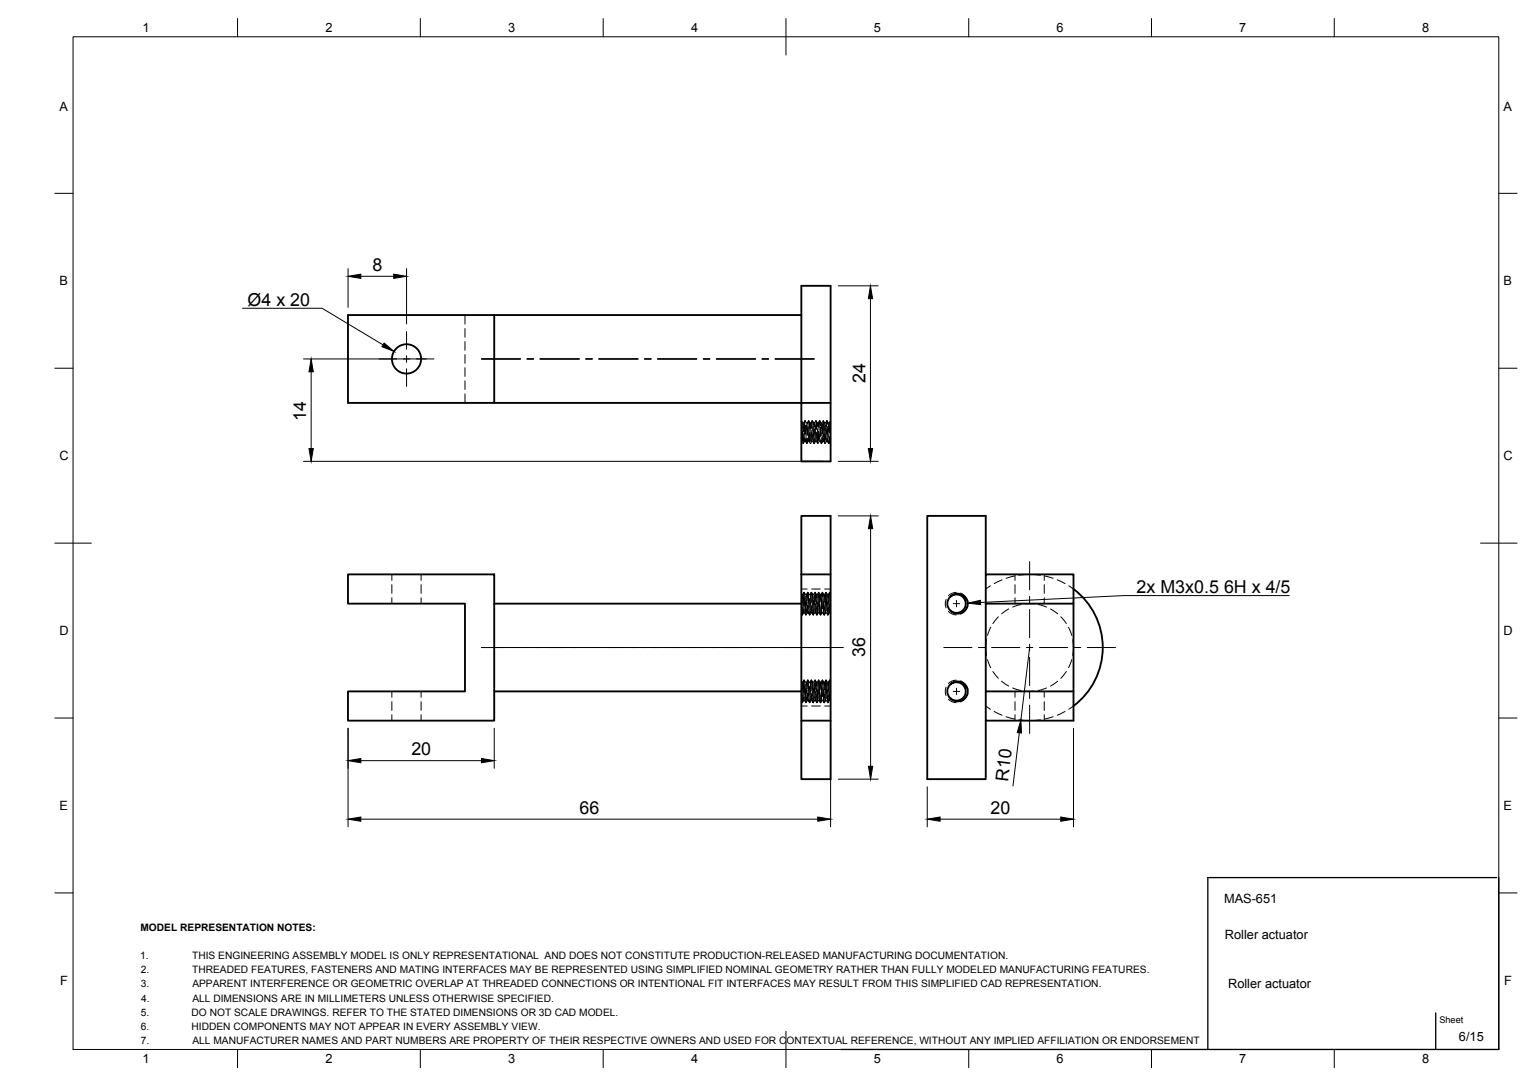
ISO-10303-21;
HEADER;
/* Generated by software containing ST-Developer
 * from STEP Tools, Inc. (www.steptools.com) 
 */

FILE_DESCRIPTION(
/* description */ ('Independent direct-acting normally-closed roller-plunger limit-switch
 CAD. Removable cover, insulated terminal supports, captured bus/conta
ct bridge, native Coil return spring, integral lower travel stop, reus
able instanced hardware and free roller. Manual geometric contact open
ing4mm; no snap-action/contact-force, electrical/current/voltage, envi
ronmental seal, safety-switch, wear, load or life certification. Exter
nal wiring and anchors omitted; fits and application engineering requi
red.'),
/* implementation_level */ '2;1');

FILE_NAME(
/* name */ 'Roller actuator.step',
/* time_stamp */ '2026-11-08T07:32:43-08:00',
/* author */ (''),
/* organization */ (''),
/* preprocessor_version */ 'ST-DEVELOPER v20.2',
/* originating_system */ 'Autodesk Translation Framework v15.17.0.0',
/* authorisation */ '');

FILE_SCHEMA (('AUTOMOTIVE_DESIGN { 1 0 10303 214 3 1 1 }'));
ENDSEC;

DATA;
#10=MECHANICAL_DESIGN_GEOMETRIC_PRESENTATION_REPRESENTATION('',(#179),#36482);
#145=SHAPE_REPRESENTATION_RELATIONSHIP('SRR','None',#36558,#162);
#162=ADVANCED_BREP_SHAPE_REPRESENTATION('',(#196),#36468);
#179=STYLED_ITEM('',(#36652),#196);
#196=MANIFOLD_SOLID_BREP('Body1',#9770);
#218=B_SPLINE_SURFACE_WITH_KNOTS('',3,3,((#21599,#21600,#21601,#21602,#21603,
#21604,#21605,#21606,#21607,#21608,#21609,#21610,#21611,#21612,#21613,#21614,
#21615,#21616,#21617,#21618,#21619,#21620,#21621,#21622,#21623,#21624,#21625,
#21626,#21627,#21628,#21629,#21630,#21631,#21632,#21633,#21634,#21635,#21636,
#21637,#21638,#21639,#21640,#21641,#21642,#21643,#21644,#21645,#21646,#21647,
#21648,#21649,#21650,#21651,#21652,#21653,#21654),(#21655,#21656,#21657,
#21658,#21659,#21660,#21661,#21662,#21663,#21664,#21665,#21666,#21667,#21668,
#21669,#21670,#21671,#21672,#21673,#21674,#21675,#21676,#21677,#21678,#21679,
#21680,#21681,#21682,#21683,#21684,#21685,#21686,#21687,#21688,#21689,#21690,
#21691,#21692,#21693,#21694,#21695,#21696,#21697,#21698,#21699,#21700,#21701,
#21702,#21703,#21704,#21705,#21706,#21707,#21708,#21709,#21710),(#21711,
#21712,#21713,#21714,#21715,#21716,#21717,#21718,#21719,#21720,#21721,#21722,
#21723,#21724,#21725,#21726,#21727,#21728,#21729,#21730,#21731,#21732,#21733,
#21734,#21735,#21736,#21737,#21738,#21739,#21740,#21741,#21742,#21743,#21744,
#21745,#21746,#21747,#21748,#21749,#21750,#21751,#21752,#21753,#21754,#21755,
#21756,#21757,#21758,#21759,#21760,#21761,#21762,#21763,#21764,#21765,#21766),
(#21767,#21768,#21769,#21770,#21771,#21772,#21773,#21774,#21775,#21776,
#21777,#21778,#21779,#21780,#21781,#21782,#21783,#21784,#21785,#21786,#21787,
#21788,#21789,#21790,#21791,#21792,#21793,#21794,#21795,#21796,#21797,#21798,
#21799,#21800,#21801,#21802,#21803,#21804,#21805,#21806,#21807,#21808,#21809,
#21810,#21811,#21812,#21813,#21814,#21815,#21816,#21817,#21818,#21819,#21820,
#21821,#21822)),.UNSPECIFIED.,.F.,.F.,.F.,(4,4),(4,1,1,1,1,1,1,1,1,1,1,
1,1,1,1,1,1,1,1,1,1,1,1,1,1,1,1,1,1,1,1,1,1,1,1,1,1,1,1,1,1,1,1,1,1,1,1,
1,1,1,1,1,1,4),(0.,0.0321584099938621),(11.8553612635793,12.8418906022433,
13.8284199409074,14.8149492795714,15.8014786182354,16.7880079568995,17.7745372955635,
18.7610666342275,19.7475959728915,20.7341253115556,21.7206546502196,22.7071839888836,
23.6937133275477,24.6802426662117,25.6667720048757,26.6533013435398,27.6398306822038,
28.6263600208678,29.6128893595319,30.5994186981959,31.5859480368599,32.5724773755239,
33.559006714188,34.545536052852,35.532065391516,36.5185947301801,37.5051240688441,
38.4916534075081,39.4781827461722,40.4647120848362,41.4512414235002,42.4377707621643,
43.4243001008283,44.4108294394923,45.3973587781563,46.3838881168204,47.3704174554844,
48.3569467941484,49.3434761328125,50.3300054714765,51.3165348101405,52.3030641488046,
53.2895934874686,54.2761228261326,55.2626521647967,56.2491815034607,57.2357108421247,
58.2222401807888,59.2087695194528,60.1952988581168,61.1818281967808,62.1683575354449,
63.1548868741089,64.1414162127729),.UNSPECIFIED.);
#219=B_SPLINE_SURFACE_WITH_KNOTS('',3,3,((#21949,#21950,#21951,#21952,#21953,
#21954,#21955,#21956,#21957,#21958,#21959,#21960,#21961,#21962,#21963,#21964,
#21965,#21966,#21967,#21968,#21969,#21970,#21971,#21972,#21973,#21974,#21975,
#21976,#21977,#21978,#21979,#21980,#21981,#21982,#21983,#21984,#21985,#21986,
#21987,#21988,#21989,#21990,#21991,#21992,#21993,#21994,#21995,#21996,#21997,
#21998,#21999,#22000,#22001,#22002,#22003,#22004),(#22005,#22006,#22007,
#22008,#22009,#22010,#22011,#22012,#22013,#22014,#22015,#22016,#22017,#22018,
#22019,#22020,#22021,#22022,#22023,#22024,#22025,#22026,#22027,#22028,#22029,
#22030,#22031,#22032,#22033,#22034,#22035,#22036,#22037,#22038,#22039,#22040,
#22041,#22042,#22043,#22044,#22045,#22046,#22047,#22048,#22049,#22050,#22051,
#22052,#22053,#22054,#22055,#22056,#22057,#22058,#22059,#22060),(#22061,
#22062,#22063,#22064,#22065,#22066,#22067,#22068,#22069,#22070,#22071,#22072,
#22073,#22074,#22075,#22076,#22077,#22078,#22079,#22080,#22081,#22082,#22083,
#22084,#22085,#22086,#22087,#22088,#22089,#22090,#22091,#22092,#22093,#22094,
#22095,#22096,#22097,#22098,#22099,#22100,#22101,#22102,#22103,#22104,#22105,
#22106,#22107,#22108,#22109,#22110,#22111,#22112,#22113,#22114,#22115,#22116),
(#22117,#22118,#22119,#22120,#22121,#22122,#22123,#22124,#22125,#22126,
#22127,#22128,#22129,#22130,#22131,#22132,#22133,#22134,#22135,#22136,#22137,
#22138,#22139,#22140,#22141,#22142,#22143,#22144,#22145,#22146,#22147,#22148,
#22149,#22150,#22151,#22152,#22153,#22154,#22155,#22156,#22157,#22158,#22159,
#22160,#22161,#22162,#22163,#22164,#22165,#22166,#22167,#22168,#22169,#22170,
#22171,#22172)),.UNSPECIFIED.,.F.,.F.,.F.,(4,4),(4,1,1,1,1,1,1,1,1,1,1,
1,1,1,1,1,1,1,1,1,1,1,1,1,1,1,1,1,1,1,1,1,1,1,1,1,1,1,1,1,1,1,1,1,1,1,1,
1,1,1,1,1,1,4),(0.,0.0321584099938621),(14.3984001269718,15.3849294656359,
16.3714588042999,17.3579881429639,18.344517481628,19.331046820292,20.317576158956,
21.30410549762,22.2906348362841,23.2771641749481,24.2636935136121,25.2502228522762,
26.2367521909402,27.2232815296042,28.2098108682683,29.1963402069323,30.1828695455963,
31.1693988842604,32.1559282229244,33.1424575615884,34.1289869002524,35.1155162389165,
36.1020455775805,37.0885749162445,38.0751042549086,39.0616335935726,40.0481629322366,
41.0346922709007,42.0212216095647,43.0077509482287,43.9942802868928,44.9808096255568,
45.9673389642208,46.9538683028848,47.9403976415489,48.9269269802129,49.9134563188769,
50.899985657541,51.886514996205,52.873044334869,53.8595736735331,54.8461030121971,
55.8326323508611,56.8191616895251,57.8056910281892,58.7922203668532,59.7787497055172,
60.7652790441813,61.7518083828453,62.7383377215093,63.7248670601734,64.7113963988374,
65.6979257375014,66.6844550761655),.UNSPECIFIED.);
#220=B_SPLINE_SURFACE_WITH_KNOTS('',3,3,((#22435,#22436,#22437,#22438,#22439,
#22440,#22441,#22442,#22443,#22444,#22445,#22446,#22447,#22448,#22449,#22450,
#22451,#22452,#22453,#22454,#22455,#22456,#22457,#22458,#22459,#22460,#22461,
#22462,#22463,#22464,#22465,#22466,#22467,#22468,#22469,#22470,#22471,#22472,
#22473,#22474,#22475,#22476,#22477,#22478,#22479,#22480,#22481,#22482,#22483,
#22484,#22485,#22486,#22487,#22488,#22489,#22490),(#22491,#22492,#22493,
#22494,#22495,#22496,#22497,#22498,#22499,#22500,#22501,#22502,#22503,#22504,
#22505,#22506,#22507,#22508,#22509,#22510,#22511,#22512,#22513,#22514,#22515,
#22516,#22517,#22518,#22519,#22520,#22521,#22522,#22523,#22524,#22525,#22526,
#22527,#22528,#22529,#22530,#22531,#22532,#22533,#22534,#22535,#22536,#22537,
#22538,#22539,#22540,#22541,#22542,#22543,#22544,#22545,#22546),(#22547,
#22548,#22549,#22550,#22551,#22552,#22553,#22554,#22555,#22556,#22557,#22558,
#22559,#22560,#22561,#22562,#22563,#22564,#22565,#22566,#22567,#22568,#22569,
#22570,#22571,#22572,#22573,#22574,#22575,#22576,#22577,#22578,#22579,#22580,
#22581,#22582,#22583,#22584,#22585,#22586,#22587,#22588,#22589,#22590,#22591,
#22592,#22593,#22594,#22595,#22596,#22597,#22598,#22599,#22600,#22601,#22602),
(#22603,#22604,#22605,#22606,#22607,#22608,#22609,#22610,#22611,#22612,
#22613,#22614,#22615,#22616,#22617,#22618,#22619,#22620,#22621,#22622,#22623,
#22624,#22625,#22626,#22627,#22628,#22629,#22630,#22631,#22632,#22633,#22634,
#22635,#22636,#22637,#22638,#22639,#22640,#22641,#22642,#22643,#22644,#22645,
#22646,#22647,#22648,#22649,#22650,#22651,#22652,#22653,#22654,#22655,#22656,
#22657,#22658)),.UNSPECIFIED.,.F.,.F.,.F.,(4,4),(4,1,1,1,1,1,1,1,1,1,1,
1,1,1,1,1,1,1,1,1,1,1,1,1,1,1,1,1,1,1,1,1,1,1,1,1,1,1,1,1,1,1,1,1,1,1,1,
1,1,1,1,1,1,4),(0.,0.0321584099938621),(11.8553612635793,12.8418906022433,
13.8284199409074,14.8149492795714,15.8014786182354,16.7880079568995,17.7745372955635,
18.7610666342275,19.7475959728915,20.7341253115556,21.7206546502196,22.7071839888836,
23.6937133275477,24.6802426662117,25.6667720048757,26.6533013435398,27.6398306822038,
28.6263600208678,29.6128893595319,30.5994186981959,31.5859480368599,32.5724773755239,
33.559006714188,34.545536052852,35.532065391516,36.5185947301801,37.5051240688441,
38.4916534075081,39.4781827461722,40.4647120848362,41.4512414235002,42.4377707621643,
43.4243001008283,44.4108294394923,45.3973587781563,46.3838881168204,47.3704174554844,
48.3569467941484,49.3434761328125,50.3300054714765,51.3165348101405,52.3030641488046,
53.2895934874686,54.2761228261326,55.2626521647967,56.2491815034607,57.2357108421247,
58.2222401807888,59.2087695194528,60.1952988581168,61.1818281967808,62.1683575354449,
63.1548868741089,64.1414162127729),.UNSPECIFIED.);
#221=B_SPLINE_SURFACE_WITH_KNOTS('',3,3,((#22733,#22734,#22735,#22736,#22737,
#22738,#22739,#22740,#22741,#22742,#22743,#22744,#22745,#22746,#22747,#22748,
#22749,#22750,#22751,#22752,#22753,#22754,#22755,#22756,#22757,#22758,#22759,
#22760,#22761,#22762,#22763,#22764,#22765,#22766,#22767,#22768,#22769,#22770,
#22771,#22772,#22773,#22774,#22775,#22776,#22777,#22778,#22779,#22780,#22781,
#22782,#22783,#22784,#22785,#22786,#22787,#22788),(#22789,#22790,#22791,
#22792,#22793,#22794,#22795,#22796,#22797,#22798,#22799,#22800,#22801,#22802,
#22803,#22804,#22805,#22806,#22807,#22808,#22809,#22810,#22811,#22812,#22813,
#22814,#22815,#22816,#22817,#22818,#22819,#22820,#22821,#22822,#22823,#22824,
#22825,#22826,#22827,#22828,#22829,#22830,#22831,#22832,#22833,#22834,#22835,
#22836,#22837,#22838,#22839,#22840,#22841,#22842,#22843,#22844),(#22845,
#22846,#22847,#22848,#22849,#22850,#22851,#22852,#22853,#22854,#22855,#22856,
#22857,#22858,#22859,#22860,#22861,#22862,#22863,#22864,#22865,#22866,#22867,
#22868,#22869,#22870,#22871,#22872,#22873,#22874,#22875,#22876,#22877,#22878,
#22879,#22880,#22881,#22882,#22883,#22884,#22885,#22886,#22887,#22888,#22889,
#22890,#22891,#22892,#22893,#22894,#22895,#22896,#22897,#22898,#22899,#22900),
(#22901,#22902,#22903,#22904,#22905,#22906,#22907,#22908,#22909,#22910,
#22911,#22912,#22913,#22914,#22915,#22916,#22917,#22918,#22919,#22920,#22921,
#22922,#22923,#22924,#22925,#22926,#22927,#22928,#22929,#22930,#22931,#22932,
#22933,#22934,#22935,#22936,#22937,#22938,#22939,#22940,#22941,#22942,#22943,
#22944,#22945,#22946,#22947,#22948,#22949,#22950,#22951,#22952,#22953,#22954,
#22955,#22956)),.UNSPECIFIED.,.F.,.F.,.F.,(4,4),(4,1,1,1,1,1,1,1,1,1,1,
1,1,1,1,1,1,1,1,1,1,1,1,1,1,1,1,1,1,1,1,1,1,1,1,1,1,1,1,1,1,1,1,1,1,1,1,
1,1,1,1,1,1,4),(0.,0.0321584099938621),(14.3984001269718,15.3849294656359,
16.3714588042999,17.3579881429639,18.344517481628,19.331046820292,20.317576158956,
21.30410549762,22.2906348362841,23.2771641749481,24.2636935136121,25.2502228522762,
26.2367521909402,27.2232815296042,28.2098108682683,29.1963402069323,30.1828695455963,
31.1693988842604,32.1559282229244,33.1424575615884,34.1289869002524,35.1155162389165,
36.1020455775805,37.0885749162445,38.0751042549086,39.0616335935726,40.0481629322366,
41.0346922709007,42.0212216095647,43.0077509482287,43.9942802868928,44.9808096255568,
45.9673389642208,46.9538683028848,47.9403976415489,48.9269269802129,49.9134563188769,
50.899985657541,51.886514996205,52.873044334869,53.8595736735331,54.8461030121971,
55.8326323508611,56.8191616895251,57.8056910281892,58.7922203668532,59.7787497055172,
60.7652790441813,61.7518083828453,62.7383377215093,63.7248670601734,64.7113963988374,
65.6979257375014,66.6844550761655),.UNSPECIFIED.);
#267=FACE_BOUND('',#1222,.T.);
#268=FACE_BOUND('',#1223,.T.);
#269=FACE_BOUND('',#1232,.T.);
#270=FACE_BOUND('',#1237,.T.);
#271=FACE_BOUND('',#1243,.T.);
#272=FACE_BOUND('',#1245,.T.);
#273=FACE_BOUND('',#1254,.T.);
#274=FACE_BOUND('',#1255,.T.);
#275=FACE_BOUND('',#1256,.T.);
#342=PLANE('',#10249);
#343=PLANE('',#10260);
#344=PLANE('',#10261);
#345=PLANE('',#10262);
#346=PLANE('',#10263);
#347=PLANE('',#10264);
#348=PLANE('',#10265);
#349=PLANE('',#10266);
#350=PLANE('',#10268);
#351=PLANE('',#10271);
#352=PLANE('',#10272);
#353=PLANE('',#10273);
#354=PLANE('',#10274);
#355=PLANE('',#10275);
#356=PLANE('',#10276);
#357=PLANE('',#10277);
#358=PLANE('',#10278);
#359=PLANE('',#10283);
#616=FACE_OUTER_BOUND('',#1186,.T.);
#617=FACE_OUTER_BOUND('',#1187,.T.);
#618=FACE_OUTER_BOUND('',#1188,.T.);
#619=FACE_OUTER_BOUND('',#1189,.T.);
#620=FACE_OUTER_BOUND('',#1190,.T.);
#621=FACE_OUTER_BOUND('',#1191,.T.);
#622=FACE_OUTER_BOUND('',#1192,.T.);
#623=FACE_OUTER_BOUND('',#1193,.T.);
#624=FACE_OUTER_BOUND('',#1194,.T.);
#625=FACE_OUTER_BOUND('',#1195,.T.);
#626=FACE_OUTER_BOUND('',#1196,.T.);
#627=FACE_OUTER_BOUND('',#1197,.T.);
#628=FACE_OUTER_BOUND('',#1198,.T.);
#629=FACE_OUTER_BOUND('',#1199,.T.);
#630=FACE_OUTER_BOUND('',#1200,.T.);
#631=FACE_OUTER_BOUND('',#1201,.T.);
#632=FACE_OUTER_BOUND('',#1202,.T.);
#633=FACE_OUTER_BOUND('',#1203,.T.);
#634=FACE_OUTER_BOUND('',#1204,.T.);
#635=FACE_OUTER_BOUND('',#1205,.T.);
#636=FACE_OUTER_BOUND('',#1206,.T.);
#637=FACE_OUTER_BOUND('',#1207,.T.);
#638=FACE_OUTER_BOUND('',#1208,.T.);
#639=FACE_OUTER_BOUND('',#1209,.T.);
#640=FACE_OUTER_BOUND('',#1210,.T.);
#641=FACE_OUTER_BOUND('',#1211,.T.);
#642=FACE_OUTER_BOUND('',#1212,.T.);
#643=FACE_OUTER_BOUND('',#1213,.T.);
#644=FACE_OUTER_BOUND('',#1214,.T.);
#645=FACE_OUTER_BOUND('',#1215,.T.);
#646=FACE_OUTER_BOUND('',#1216,.T.);
#647=FACE_OUTER_BOUND('',#1217,.T.);
#648=FACE_OUTER_BOUND('',#1218,.T.);
#649=FACE_OUTER_BOUND('',#1219,.T.);
#650=FACE_OUTER_BOUND('',#1220,.T.);
#651=FACE_OUTER_BOUND('',#1221,.T.);
#652=FACE_OUTER_BOUND('',#1224,.T.);
#653=FACE_OUTER_BOUND('',#1225,.T.);
#654=FACE_OUTER_BOUND('',#1226,.T.);
#655=FACE_OUTER_BOUND('',#1227,.T.);
#656=FACE_OUTER_BOUND('',#1228,.T.);
#657=FACE_OUTER_BOUND('',#1229,.T.);
#658=FACE_OUTER_BOUND('',#1230,.T.);
#659=FACE_OUTER_BOUND('',#1231,.T.);
#660=FACE_OUTER_BOUND('',#1233,.T.);
#661=FACE_OUTER_BOUND('',#1234,.T.);
#662=FACE_OUTER_BOUND('',#1235,.T.);
#663=FACE_OUTER_BOUND('',#1236,.T.);
#664=FACE_OUTER_BOUND('',#1238,.T.);
#665=FACE_OUTER_BOUND('',#1239,.T.);
#666=FACE_OUTER_BOUND('',#1240,.T.);
#667=FACE_OUTER_BOUND('',#1241,.T.);
#668=FACE_OUTER_BOUND('',#1242,.T.);
#669=FACE_OUTER_BOUND('',#1244,.T.);
#670=FACE_OUTER_BOUND('',#1246,.T.);
#671=FACE_OUTER_BOUND('',#1247,.T.);
#672=FACE_OUTER_BOUND('',#1248,.T.);
#673=FACE_OUTER_BOUND('',#1249,.T.);
#674=FACE_OUTER_BOUND('',#1250,.T.);
#675=FACE_OUTER_BOUND('',#1251,.T.);
#676=FACE_OUTER_BOUND('',#1252,.T.);
#677=FACE_OUTER_BOUND('',#1253,.T.);
#1186=EDGE_LOOP('',(#6952,#6953,#6954,#6955));
#1187=EDGE_LOOP('',(#6956,#6957,#6958,#6959));
#1188=EDGE_LOOP('',(#6960,#6961,#6962,#6963));
#1189=EDGE_LOOP('',(#6964,#6965,#6966,#6967));
#1190=EDGE_LOOP('',(#6968,#6969,#6970,#6971));
#1191=EDGE_LOOP('',(#6972,#6973,#6974,#6975));
#1192=EDGE_LOOP('',(#6976,#6977,#6978,#6979));
#1193=EDGE_LOOP('',(#6980,#6981,#6982,#6983));
#1194=EDGE_LOOP('',(#6984,#6985,#6986,#6987));
#1195=EDGE_LOOP('',(#6988,#6989,#6990,#6991));
#1196=EDGE_LOOP('',(#6992,#6993,#6994,#6995));
#1197=EDGE_LOOP('',(#6996,#6997,#6998,#6999));
#1198=EDGE_LOOP('',(#7000,#7001,#7002,#7003));
#1199=EDGE_LOOP('',(#7004,#7005,#7006,#7007));
#1200=EDGE_LOOP('',(#7008,#7009,#7010,#7011));
#1201=EDGE_LOOP('',(#7012,#7013,#7014,#7015));
#1202=EDGE_LOOP('',(#7016,#7017,#7018,#7019));
#1203=EDGE_LOOP('',(#7020,#7021,#7022,#7023));
#1204=EDGE_LOOP('',(#7024,#7025,#7026,#7027));
#1205=EDGE_LOOP('',(#7028,#7029,#7030,#7031));
#1206=EDGE_LOOP('',(#7032,#7033,#7034,#7035));
#1207=EDGE_LOOP('',(#7036,#7037,#7038,#7039));
#1208=EDGE_LOOP('',(#7040,#7041,#7042,#7043));
#1209=EDGE_LOOP('',(#7044,#7045,#7046,#7047));
#1210=EDGE_LOOP('',(#7048,#7049,#7050,#7051));
#1211=EDGE_LOOP('',(#7052,#7053,#7054,#7055));
#1212=EDGE_LOOP('',(#7056,#7057,#7058,#7059));
#1213=EDGE_LOOP('',(#7060,#7061,#7062,#7063));
#1214=EDGE_LOOP('',(#7064,#7065,#7066,#7067));
#1215=EDGE_LOOP('',(#7068,#7069,#7070,#7071));
#1216=EDGE_LOOP('',(#7072,#7073,#7074,#7075));
#1217=EDGE_LOOP('',(#7076,#7077,#7078,#7079));
#1218=EDGE_LOOP('',(#7080,#7081,#7082,#7083));
#1219=EDGE_LOOP('',(#7084,#7085,#7086,#7087,#7088,#7089,#7090,#7091,#7092,
#7093,#7094,#7095,#7096,#7097,#7098,#7099,#7100,#7101,#7102,#7103));
#1220=EDGE_LOOP('',(#7104,#7105,#7106,#7107,#7108,#7109,#7110,#7111,#7112,
#7113,#7114,#7115,#7116,#7117,#7118,#7119,#7120,#7121,#7122,#7123));
#1221=EDGE_LOOP('',(#7124,#7125,#7126,#7127,#7128,#7129));
#1222=EDGE_LOOP('',(#7130,#7131,#7132,#7133));
#1223=EDGE_LOOP('',(#7134,#7135,#7136,#7137));
#1224=EDGE_LOOP('',(#7138,#7139,#7140,#7141));
#1225=EDGE_LOOP('',(#7142,#7143,#7144,#7145,#7146,#7147,#7148,#7149,#7150,
#7151,#7152,#7153,#7154,#7155,#7156,#7157,#7158,#7159,#7160,#7161));
#1226=EDGE_LOOP('',(#7162,#7163,#7164,#7165,#7166,#7167,#7168,#7169,#7170,
#7171,#7172,#7173,#7174,#7175,#7176,#7177,#7178,#7179,#7180,#7181));
#1227=EDGE_LOOP('',(#7182,#7183,#7184,#7185));
#1228=EDGE_LOOP('',(#7186,#7187,#7188,#7189));
#1229=EDGE_LOOP('',(#7190,#7191,#7192,#7193));
#1230=EDGE_LOOP('',(#7194,#7195,#7196,#7197));
#1231=EDGE_LOOP('',(#7198,#7199,#7200,#7201));
#1232=EDGE_LOOP('',(#7202));
#1233=EDGE_LOOP('',(#7203,#7204,#7205,#7206));
#1234=EDGE_LOOP('',(#7207,#7208,#7209,#7210,#7211,#7212,#7213,#7214,#7215));
#1235=EDGE_LOOP('',(#7216,#7217,#7218,#7219));
#1236=EDGE_LOOP('',(#7220,#7221,#7222,#7223));
#1237=EDGE_LOOP('',(#7224));
#1238=EDGE_LOOP('',(#7225,#7226,#7227,#7228));
#1239=EDGE_LOOP('',(#7229,#7230,#7231,#7232));
#1240=EDGE_LOOP('',(#7233,#7234,#7235,#7236,#7237));
#1241=EDGE_LOOP('',(#7238,#7239,#7240,#7241,#7242,#7243,#7244,#7245,#7246));
#1242=EDGE_LOOP('',(#7247,#7248,#7249,#7250));
#1243=EDGE_LOOP('',(#7251));
#1244=EDGE_LOOP('',(#7252,#7253,#7254,#7255));
#1245=EDGE_LOOP('',(#7256));
#1246=EDGE_LOOP('',(#7257,#7258,#7259,#7260));
#1247=EDGE_LOOP('',(#7261,#7262,#7263,#7264));
#1248=EDGE_LOOP('',(#7265,#7266,#7267,#7268));
#1249=EDGE_LOOP('',(#7269,#7270,#7271,#7272));
#1250=EDGE_LOOP('',(#7273,#7274,#7275,#7276));
#1251=EDGE_LOOP('',(#7277,#7278,#7279,#7280));
#1252=EDGE_LOOP('',(#7281,#7282,#7283,#7284,#7285,#7286));
#1253=EDGE_LOOP('',(#7287,#7288,#7289,#7290,#7291,#7292));
#1254=EDGE_LOOP('',(#7293,#7294,#7295,#7296));
#1255=EDGE_LOOP('',(#7297,#7298,#7299,#7300));
#1256=EDGE_LOOP('',(#7301));
#1644=CIRCLE('',#10209,0.12645);
#1645=CIRCLE('',#10217,0.12645);
#1646=CIRCLE('',#10219,0.12645);
#1647=CIRCLE('',#10227,0.12645);
#1648=CIRCLE('',#10229,0.1543);
#1649=CIRCLE('',#10237,0.1543);
#1650=CIRCLE('',#10239,0.1543);
#1651=CIRCLE('',#10247,0.1543);
#1652=CIRCLE('',#10250,1.);
#1653=CIRCLE('',#10255,0.2);
#1654=CIRCLE('',#10256,0.2);
#1655=CIRCLE('',#10258,0.2);
#1656=CIRCLE('',#10259,0.2);
#1657=CIRCLE('',#10267,0.6);
#1658=CIRCLE('',#10269,0.6);
#1659=CIRCLE('',#10270,0.6);
#1660=CIRCLE('',#10280,1.);
#1661=CIRCLE('',#10282,0.6);
#1974=B_SPLINE_CURVE_WITH_KNOTS('',3,(#20484,#20485,#20486,#20487),
 .UNSPECIFIED.,.F.,.F.,(4,4),(51.5750455984138,52.2860549491936),
 .UNSPECIFIED.);
#1975=B_SPLINE_CURVE_WITH_KNOTS('',3,(#20490,#20491,#20492,#20493,#20494,
#20495,#20496,#20497,#20498,#20499),.UNSPECIFIED.,.F.,.F.,(4,3,3,4),(-50.2654824574367,
-49.3264669332015,-48.3399375945375,-47.8348991546268),.UNSPECIFIED.);
#1976=B_SPLINE_CURVE_WITH_KNOTS('',3,(#20504,#20505,#20506,#20507,#20508,
#20509,#20510,#20511,#20512,#20513,#20514,#20515,#20516,#20517,#20518,#20519,
#20520,#20521,#20522,#20523,#20524,#20525,#20526,#20527,#20528),
 .UNSPECIFIED.,.F.,.F.,(4,3,3,3,3,3,3,3,4),(45.2918602912342,45.3803495785454,
46.3668789172094,47.3534082558735,48.3399375945375,49.3264669332015,50.3129962718656,
51.2995256105296,51.5750455984138),.UNSPECIFIED.);
#1977=B_SPLINE_CURVE_WITH_KNOTS('',3,(#20529,#20530,#20531,#20532,#20533,
#20534,#20535,#20536,#20537,#20538,#20539,#20540,#20541,#20542,#20543,#20544,
#20545,#20546,#20547,#20548,#20549,#20550),.UNSPECIFIED.,.F.,.F.,(4,3,3,
3,3,3,3,4),(-47.8348991546268,-47.3534082558735,-46.3668789172095,-45.3803495785454,
-44.3938202398814,-43.4072909012174,-42.4207615625533,-41.5517138474472),
 .UNSPECIFIED.);
#1978=B_SPLINE_CURVE_WITH_KNOTS('',3,(#20555,#20556,#20557,#20558,#20559,
#20560,#20561,#20562,#20563,#20564,#20565,#20566,#20567,#20568,#20569,#20570,
#20571,#20572,#20573,#20574,#20575,#20576),.UNSPECIFIED.,.F.,.F.,(4,3,3,
3,3,3,3,4),(39.0086749840546,39.4611735465612,40.4477028852253,41.4342322238893,
42.4207615625533,43.4072909012174,44.3938202398814,45.2918602912342),
 .UNSPECIFIED.);
#1979=B_SPLINE_CURVE_WITH_KNOTS('',3,(#20577,#20578,#20579,#20580,#20581,
#20582,#20583,#20584,#20585,#20586,#20587,#20588,#20589,#20590,#20591,#20592,
#20593,#20594,#20595,#20596,#20597,#20598,#20599,#20600,#20601),
 .UNSPECIFIED.,.F.,.F.,(4,3,3,3,3,3,3,3,4),(-41.5517138474472,-41.4342322238893,
-40.4477028852253,-39.4611735465612,-38.4746442078972,-37.4881148692332,
-36.5015855305691,-35.5150561919051,-35.2685285402676),.UNSPECIFIED.);
#1980=B_SPLINE_CURVE_WITH_KNOTS('',3,(#20606,#20607,#20608,#20609,#20610,
#20611,#20612,#20613,#20614,#20615,#20616,#20617,#20618,#20619,#20620,#20621,
#20622,#20623,#20624,#20625,#20626,#20627),.UNSPECIFIED.,.F.,.F.,(4,3,3,
3,3,3,3,4),(32.725489676875,33.541997514577,34.5285268532411,35.5150561919051,
36.5015855305691,37.4881148692332,38.4746442078972,39.0086749840546),
 .UNSPECIFIED.);
#1981=B_SPLINE_CURVE_WITH_KNOTS('',3,(#20628,#20629,#20630,#20631,#20632,
#20633,#20634,#20635,#20636,#20637,#20638,#20639,#20640,#20641,#20642,#20643,
#20644,#20645,#20646,#20647,#20648,#20649),.UNSPECIFIED.,.F.,.F.,(4,3,3,
3,3,3,3,4),(-35.2685285402676,-34.5285268532411,-33.541997514577,-32.555468175913,
-31.568938837249,-30.582409498585,-29.5958801599209,-28.985343233088),
 .UNSPECIFIED.);
#1982=B_SPLINE_CURVE_WITH_KNOTS('',3,(#20654,#20655,#20656,#20657,#20658,
#20659,#20660,#20661,#20662,#20663,#20664,#20665,#20666,#20667,#20668,#20669,
#20670,#20671,#20672,#20673,#20674,#20675,#20676,#20677,#20678),
 .UNSPECIFIED.,.F.,.F.,(4,3,3,3,3,3,3,3,4),(26.4423043696954,26.6362921439288,
27.6228214825929,28.6093508212569,29.5958801599209,30.582409498585,31.568938837249,
32.555468175913,32.725489676875),.UNSPECIFIED.);
#1983=B_SPLINE_CURVE_WITH_KNOTS('',3,(#20679,#20680,#20681,#20682,#20683,
#20684,#20685,#20686,#20687,#20688,#20689,#20690,#20691,#20692,#20693,#20694,
#20695,#20696,#20697,#20698,#20699,#20700),.UNSPECIFIED.,.F.,.F.,(4,3,3,
3,3,3,3,4),(-28.985343233088,-28.6093508212569,-27.6228214825929,-26.6362921439288,
-25.6497628052648,-24.6632334666008,-23.6767041279367,-22.7021579259084),
 .UNSPECIFIED.);
#1984=B_SPLINE_CURVE_WITH_KNOTS('',3,(#20705,#20706,#20707,#20708,#20709,
#20710,#20711,#20712,#20713,#20714,#20715,#20716,#20717,#20718,#20719,#20720,
#20721,#20722,#20723,#20724,#20725,#20726),.UNSPECIFIED.,.F.,.F.,(4,3,3,
3,3,3,3,4),(20.1591190625159,20.7171161119446,21.7036454506087,22.6901747892727,
23.6767041279367,24.6632334666008,25.6497628052648,26.4423043696954),
 .UNSPECIFIED.);
#1985=B_SPLINE_CURVE_WITH_KNOTS('',3,(#20727,#20728,#20729,#20730,#20731,
#20732,#20733,#20734,#20735,#20736,#20737,#20738,#20739,#20740,#20741,#20742,
#20743,#20744,#20745,#20746,#20747,#20748,#20749,#20750,#20751),
 .UNSPECIFIED.,.F.,.F.,(4,3,3,3,3,3,3,3,4),(-22.7021579259084,-22.6901747892727,
-21.7036454506087,-20.7171161119446,-19.7305867732806,-18.7440574346166,
-17.7575280959526,-16.7709987572885,-16.4189726187288),.UNSPECIFIED.);
#1986=B_SPLINE_CURVE_WITH_KNOTS('',3,(#20756,#20757,#20758,#20759,#20760,
#20761,#20762,#20763,#20764,#20765,#20766,#20767,#20768,#20769,#20770,#20771,
#20772,#20773,#20774,#20775,#20776,#20777),.UNSPECIFIED.,.F.,.F.,(4,3,3,
3,3,3,3,4),(13.8759337553363,14.7979400799605,15.7844694186245,16.7709987572885,
17.7575280959526,18.7440574346166,19.7305867732806,20.1591190625159),
 .UNSPECIFIED.);
#1987=B_SPLINE_CURVE_WITH_KNOTS('',3,(#20778,#20779,#20780,#20781,#20782,
#20783,#20784,#20785,#20786,#20787,#20788,#20789,#20790,#20791,#20792,#20793,
#20794,#20795,#20796,#20797,#20798,#20799),.UNSPECIFIED.,.F.,.F.,(4,3,3,
3,3,3,3,4),(-16.4189726187288,-15.7844694186245,-14.7979400799605,-13.8114107412964,
-12.8248814026324,-11.8383520639684,-10.8518227253043,-10.1357873115492),
 .UNSPECIFIED.);
#1988=B_SPLINE_CURVE_WITH_KNOTS('',3,(#20805,#20806,#20807,#20808,#20809,
#20810,#20811,#20812,#20813,#20814,#20815,#20816,#20817),.UNSPECIFIED.,
 .F.,.F.,(4,3,3,3,4),(-3.85260200436966,-2.95958801599209,-1.97305867732806,
-0.986529338664031,0.),.UNSPECIFIED.);
#1989=B_SPLINE_CURVE_WITH_KNOTS('',3,(#20820,#20821,#20822,#20823,#20824,
#20825,#20826,#20827,#20828,#20829,#20830,#20831,#20832,#20833,#20834,#20835,
#20836,#20837,#20838),.UNSPECIFIED.,.F.,.F.,(4,3,3,3,3,3,4),(2.0205724917569,
2.95958801599209,3.94611735465613,4.93264669332016,5.91917603198418,6.90570537064821,
7.5927484481567),.UNSPECIFIED.);
#1990=B_SPLINE_CURVE_WITH_KNOTS('',3,(#20844,#20845,#20846,#20847),
 .UNSPECIFIED.,.F.,.F.,(4,4),(51.5750455984138,52.2860549491936),
 .UNSPECIFIED.);
#1991=B_SPLINE_CURVE_WITH_KNOTS('',3,(#20850,#20851,#20852,#20853,#20854,
#20855,#20856,#20857,#20858,#20859),.UNSPECIFIED.,.F.,.F.,(4,3,3,4),(-50.2654824574367,
-49.3264669332015,-48.3399375945375,-47.8348991546268),.UNSPECIFIED.);
#1992=B_SPLINE_CURVE_WITH_KNOTS('',3,(#20864,#20865,#20866,#20867,#20868,
#20869,#20870,#20871,#20872,#20873,#20874,#20875,#20876,#20877,#20878,#20879,
#20880,#20881,#20882,#20883,#20884,#20885,#20886,#20887,#20888),
 .UNSPECIFIED.,.F.,.F.,(4,3,3,3,3,3,3,3,4),(45.2918602912342,45.3803495785454,
46.3668789172094,47.3534082558735,48.3399375945375,49.3264669332015,50.3129962718656,
51.2995256105296,51.5750455984138),.UNSPECIFIED.);
#1993=B_SPLINE_CURVE_WITH_KNOTS('',3,(#20889,#20890,#20891,#20892,#20893,
#20894,#20895,#20896,#20897,#20898,#20899,#20900,#20901,#20902,#20903,#20904,
#20905,#20906,#20907,#20908,#20909,#20910),.UNSPECIFIED.,.F.,.F.,(4,3,3,
3,3,3,3,4),(-47.8348991546268,-47.3534082558735,-46.3668789172095,-45.3803495785454,
-44.3938202398814,-43.4072909012174,-42.4207615625533,-41.5517138474472),
 .UNSPECIFIED.);
#1994=B_SPLINE_CURVE_WITH_KNOTS('',3,(#20915,#20916,#20917,#20918,#20919,
#20920,#20921,#20922,#20923,#20924,#20925,#20926,#20927,#20928,#20929,#20930,
#20931,#20932,#20933,#20934,#20935,#20936),.UNSPECIFIED.,.F.,.F.,(4,3,3,
3,3,3,3,4),(39.0086749840546,39.4611735465612,40.4477028852253,41.4342322238893,
42.4207615625533,43.4072909012174,44.3938202398814,45.2918602912342),
 .UNSPECIFIED.);
#1995=B_SPLINE_CURVE_WITH_KNOTS('',3,(#20937,#20938,#20939,#20940,#20941,
#20942,#20943,#20944,#20945,#20946,#20947,#20948,#20949,#20950,#20951,#20952,
#20953,#20954,#20955,#20956,#20957,#20958,#20959,#20960,#20961),
 .UNSPECIFIED.,.F.,.F.,(4,3,3,3,3,3,3,3,4),(-41.5517138474472,-41.4342322238893,
-40.4477028852253,-39.4611735465612,-38.4746442078972,-37.4881148692332,
-36.5015855305691,-35.5150561919051,-35.2685285402676),.UNSPECIFIED.);
#1996=B_SPLINE_CURVE_WITH_KNOTS('',3,(#20966,#20967,#20968,#20969,#20970,
#20971,#20972,#20973,#20974,#20975,#20976,#20977,#20978,#20979,#20980,#20981,
#20982,#20983,#20984,#20985,#20986,#20987),.UNSPECIFIED.,.F.,.F.,(4,3,3,
3,3,3,3,4),(32.725489676875,33.541997514577,34.5285268532411,35.5150561919051,
36.5015855305691,37.4881148692332,38.4746442078972,39.0086749840546),
 .UNSPECIFIED.);
#1997=B_SPLINE_CURVE_WITH_KNOTS('',3,(#20988,#20989,#20990,#20991,#20992,
#20993,#20994,#20995,#20996,#20997,#20998,#20999,#21000,#21001,#21002,#21003,
#21004,#21005,#21006,#21007,#21008,#21009),.UNSPECIFIED.,.F.,.F.,(4,3,3,
3,3,3,3,4),(-35.2685285402676,-34.5285268532411,-33.541997514577,-32.555468175913,
-31.568938837249,-30.582409498585,-29.5958801599209,-28.985343233088),
 .UNSPECIFIED.);
#1998=B_SPLINE_CURVE_WITH_KNOTS('',3,(#21014,#21015,#21016,#21017,#21018,
#21019,#21020,#21021,#21022,#21023,#21024,#21025,#21026,#21027,#21028,#21029,
#21030,#21031,#21032,#21033,#21034,#21035,#21036,#21037,#21038),
 .UNSPECIFIED.,.F.,.F.,(4,3,3,3,3,3,3,3,4),(26.4423043696954,26.6362921439288,
27.6228214825929,28.6093508212569,29.5958801599209,30.582409498585,31.568938837249,
32.555468175913,32.725489676875),.UNSPECIFIED.);
#1999=B_SPLINE_CURVE_WITH_KNOTS('',3,(#21039,#21040,#21041,#21042,#21043,
#21044,#21045,#21046,#21047,#21048,#21049,#21050,#21051,#21052,#21053,#21054,
#21055,#21056,#21057,#21058,#21059,#21060),.UNSPECIFIED.,.F.,.F.,(4,3,3,
3,3,3,3,4),(-28.985343233088,-28.6093508212569,-27.6228214825929,-26.6362921439288,
-25.6497628052648,-24.6632334666008,-23.6767041279367,-22.7021579259084),
 .UNSPECIFIED.);
#2000=B_SPLINE_CURVE_WITH_KNOTS('',3,(#21065,#21066,#21067,#21068,#21069,
#21070,#21071,#21072,#21073,#21074,#21075,#21076,#21077,#21078,#21079,#21080,
#21081,#21082,#21083,#21084,#21085,#21086),.UNSPECIFIED.,.F.,.F.,(4,3,3,
3,3,3,3,4),(20.1591190625159,20.7171161119446,21.7036454506087,22.6901747892727,
23.6767041279367,24.6632334666008,25.6497628052648,26.4423043696954),
 .UNSPECIFIED.);
#2001=B_SPLINE_CURVE_WITH_KNOTS('',3,(#21087,#21088,#21089,#21090,#21091,
#21092,#21093,#21094,#21095,#21096,#21097,#21098,#21099,#21100,#21101,#21102,
#21103,#21104,#21105,#21106,#21107,#21108,#21109,#21110,#21111),
 .UNSPECIFIED.,.F.,.F.,(4,3,3,3,3,3,3,3,4),(-22.7021579259084,-22.6901747892727,
-21.7036454506087,-20.7171161119446,-19.7305867732806,-18.7440574346166,
-17.7575280959526,-16.7709987572885,-16.4189726187288),.UNSPECIFIED.);
#2002=B_SPLINE_CURVE_WITH_KNOTS('',3,(#21116,#21117,#21118,#21119,#21120,
#21121,#21122,#21123,#21124,#21125,#21126,#21127,#21128,#21129,#21130,#21131,
#21132,#21133,#21134,#21135,#21136,#21137),.UNSPECIFIED.,.F.,.F.,(4,3,3,
3,3,3,3,4),(13.8759337553363,14.7979400799605,15.7844694186245,16.7709987572885,
17.7575280959526,18.7440574346166,19.7305867732806,20.1591190625159),
 .UNSPECIFIED.);
#2003=B_SPLINE_CURVE_WITH_KNOTS('',3,(#21138,#21139,#21140,#21141,#21142,
#21143,#21144,#21145,#21146,#21147,#21148,#21149,#21150,#21151,#21152,#21153,
#21154,#21155,#21156,#21157,#21158,#21159),.UNSPECIFIED.,.F.,.F.,(4,3,3,
3,3,3,3,4),(-16.4189726187288,-15.7844694186245,-14.7979400799605,-13.8114107412964,
-12.8248814026324,-11.8383520639684,-10.8518227253043,-10.1357873115492),
 .UNSPECIFIED.);
#2004=B_SPLINE_CURVE_WITH_KNOTS('',3,(#21165,#21166,#21167,#21168,#21169,
#21170,#21171,#21172,#21173,#21174,#21175,#21176,#21177),.UNSPECIFIED.,
 .F.,.F.,(4,3,3,3,4),(-3.85260200436966,-2.95958801599209,-1.97305867732806,
-0.986529338664031,0.),.UNSPECIFIED.);
#2005=B_SPLINE_CURVE_WITH_KNOTS('',3,(#21180,#21181,#21182,#21183,#21184,
#21185,#21186,#21187,#21188,#21189,#21190,#21191,#21192,#21193,#21194,#21195,
#21196,#21197,#21198),.UNSPECIFIED.,.F.,.F.,(4,3,3,3,3,3,4),(2.0205724917569,
2.95958801599209,3.94611735465612,4.93264669332016,5.91917603198418,6.90570537064822,
7.5927484481567),.UNSPECIFIED.);
#2006=B_SPLINE_CURVE_WITH_KNOTS('',3,(#21204,#21205,#21206,#21207,#21208,
#21209,#21210,#21211),.UNSPECIFIED.,.F.,.F.,(4,1,1,1,1,4),(59.6902604182061,
60.1952988581168,61.1818281967808,62.1683575354449,63.1548868741089,64.1414162127729),
 .UNSPECIFIED.);
#2007=B_SPLINE_CURVE_WITH_KNOTS('',3,(#21214,#21215,#21216,#21217,#21218,
#21219,#21220,#21221,#21222),.UNSPECIFIED.,.F.,.F.,(4,1,1,1,1,1,4),(59.6902604182061,
59.7787497055172,60.7652790441813,61.7518083828453,62.7383377215093,63.7248670601734,
64.6638825844086),.UNSPECIFIED.);
#2008=B_SPLINE_CURVE_WITH_KNOTS('',3,(#21227,#21228,#21229,#21230,#21231,
#21232,#21233,#21234,#21235,#21236),.UNSPECIFIED.,.F.,.F.,(4,1,1,1,1,1,
1,4),(53.4070751110265,54.2761228261326,55.2626521647967,56.2491815034607,
57.2357108421247,58.2222401807888,59.2087695194528,59.6902604182061),
 .UNSPECIFIED.);
#2009=B_SPLINE_CURVE_WITH_KNOTS('',3,(#21237,#21238,#21239,#21240,#21241,
#21242,#21243,#21244,#21245,#21246),.UNSPECIFIED.,.F.,.F.,(4,1,1,1,1,1,
1,4),(53.4070751110265,53.8595736735331,54.8461030121971,55.8326323508611,
56.8191616895251,57.8056910281892,58.7922203668532,59.6902604182061),
 .UNSPECIFIED.);
#2010=B_SPLINE_CURVE_WITH_KNOTS('',3,(#21251,#21252,#21253,#21254,#21255,
#21256,#21257,#21258,#21259,#21260,#21261),.UNSPECIFIED.,.F.,.F.,(4,1,1,
1,1,1,1,1,4),(47.1238898038469,47.3704174554844,48.3569467941484,49.3434761328125,
50.3300054714765,51.3165348101405,52.3030641488046,53.2895934874686,53.4070751110265),
 .UNSPECIFIED.);
#2011=B_SPLINE_CURVE_WITH_KNOTS('',3,(#21262,#21263,#21264,#21265,#21266,
#21267,#21268,#21269,#21270,#21271),.UNSPECIFIED.,.F.,.F.,(4,1,1,1,1,1,
1,4),(47.1238898038469,47.9403976415489,48.9269269802129,49.9134563188769,
50.899985657541,51.886514996205,52.873044334869,53.4070751110265),
 .UNSPECIFIED.);
#2012=B_SPLINE_CURVE_WITH_KNOTS('',3,(#21276,#21277,#21278,#21279,#21280,
#21281,#21282,#21283,#21284,#21285),.UNSPECIFIED.,.F.,.F.,(4,1,1,1,1,1,
1,4),(40.8407044966673,41.4512414235002,42.4377707621643,43.4243001008283,
44.4108294394923,45.3973587781563,46.3838881168204,47.1238898038469),
 .UNSPECIFIED.);
#2013=B_SPLINE_CURVE_WITH_KNOTS('',3,(#21286,#21287,#21288,#21289,#21290,
#21291,#21292,#21293,#21294,#21295,#21296),.UNSPECIFIED.,.F.,.F.,(4,1,1,
1,1,1,1,1,4),(40.8407044966673,41.0346922709007,42.0212216095647,43.0077509482287,
43.9942802868928,44.9808096255568,45.9673389642208,46.9538683028848,47.1238898038469),
 .UNSPECIFIED.);
#2014=B_SPLINE_CURVE_WITH_KNOTS('',3,(#21301,#21302,#21303,#21304,#21305,
#21306,#21307,#21308,#21309,#21310),.UNSPECIFIED.,.F.,.F.,(4,1,1,1,1,1,
1,4),(34.5575191894877,35.532065391516,36.5185947301801,37.5051240688441,
38.4916534075081,39.4781827461722,40.4647120848362,40.8407044966673),
 .UNSPECIFIED.);
#2015=B_SPLINE_CURVE_WITH_KNOTS('',3,(#21311,#21312,#21313,#21314,#21315,
#21316,#21317,#21318,#21319,#21320),.UNSPECIFIED.,.F.,.F.,(4,1,1,1,1,1,
1,4),(34.5575191894877,35.1155162389165,36.1020455775805,37.0885749162445,
38.0751042549086,39.0616335935726,40.0481629322366,40.8407044966673),
 .UNSPECIFIED.);
#2016=B_SPLINE_CURVE_WITH_KNOTS('',3,(#21325,#21326,#21327,#21328,#21329,
#21330,#21331,#21332,#21333,#21334,#21335),.UNSPECIFIED.,.F.,.F.,(4,1,1,
1,1,1,1,1,4),(28.2743338823081,28.6263600208678,29.6128893595319,30.5994186981959,
31.5859480368599,32.5724773755239,33.559006714188,34.545536052852,34.5575191894877),
 .UNSPECIFIED.);
#2017=B_SPLINE_CURVE_WITH_KNOTS('',3,(#21336,#21337,#21338,#21339,#21340,
#21341,#21342,#21343,#21344,#21345),.UNSPECIFIED.,.F.,.F.,(4,1,1,1,1,1,
1,4),(28.2743338823081,29.1963402069323,30.1828695455963,31.1693988842604,
32.1559282229244,33.1424575615884,34.1289869002524,34.5575191894877),
 .UNSPECIFIED.);
#2018=B_SPLINE_CURVE_WITH_KNOTS('',3,(#21350,#21351,#21352,#21353,#21354,
#21355,#21356,#21357,#21358,#21359),.UNSPECIFIED.,.F.,.F.,(4,1,1,1,1,1,
1,4),(21.9911485751285,22.7071839888836,23.6937133275477,24.6802426662117,
25.6667720048757,26.6533013435398,27.6398306822038,28.2743338823081),
 .UNSPECIFIED.);
#2019=B_SPLINE_CURVE_WITH_KNOTS('',3,(#21360,#21361,#21362,#21363,#21364,
#21365,#21366,#21367,#21368,#21369,#21370),.UNSPECIFIED.,.F.,.F.,(4,1,1,
1,1,1,1,1,4),(21.9911485751285,22.2906348362841,23.2771641749481,24.2636935136121,
25.2502228522762,26.2367521909402,27.2232815296042,28.2098108682683,28.2743338823081),
 .UNSPECIFIED.);
#2020=B_SPLINE_CURVE_WITH_KNOTS('',3,(#21376,#21377,#21378,#21379,#21380),
 .UNSPECIFIED.,.F.,.F.,(4,1,4),(14.3984001269718,15.3849294656359,15.707963267949),
 .UNSPECIFIED.);
#2021=B_SPLINE_CURVE_WITH_KNOTS('',3,(#21383,#21384,#21385,#21386,#21387),
 .UNSPECIFIED.,.F.,.F.,(4,1,4),(13.8759337553362,14.8149492795714,15.7079632679489),
 .UNSPECIFIED.);
#2022=B_SPLINE_CURVE_WITH_KNOTS('',3,(#21393,#21394,#21395,#21396,#21397,
#21398,#21399,#21400),.UNSPECIFIED.,.F.,.F.,(4,1,1,1,1,4),(59.6902604182061,
60.1952988581168,61.1818281967808,62.1683575354449,63.1548868741089,64.1414162127729),
 .UNSPECIFIED.);
#2023=B_SPLINE_CURVE_WITH_KNOTS('',3,(#21403,#21404,#21405,#21406,#21407,
#21408,#21409,#21410,#21411),.UNSPECIFIED.,.F.,.F.,(4,1,1,1,1,1,4),(59.6902604182061,
59.7787497055172,60.7652790441813,61.7518083828453,62.7383377215093,63.7248670601734,
64.6638825844086),.UNSPECIFIED.);
#2024=B_SPLINE_CURVE_WITH_KNOTS('',3,(#21416,#21417,#21418,#21419,#21420,
#21421,#21422,#21423,#21424,#21425),.UNSPECIFIED.,.F.,.F.,(4,1,1,1,1,1,
1,4),(53.4070751110265,54.2761228261326,55.2626521647967,56.2491815034607,
57.2357108421247,58.2222401807888,59.2087695194528,59.6902604182061),
 .UNSPECIFIED.);
#2025=B_SPLINE_CURVE_WITH_KNOTS('',3,(#21426,#21427,#21428,#21429,#21430,
#21431,#21432,#21433,#21434,#21435),.UNSPECIFIED.,.F.,.F.,(4,1,1,1,1,1,
1,4),(53.4070751110265,53.8595736735331,54.8461030121971,55.8326323508611,
56.8191616895251,57.8056910281892,58.7922203668532,59.6902604182061),
 .UNSPECIFIED.);
#2026=B_SPLINE_CURVE_WITH_KNOTS('',3,(#21440,#21441,#21442,#21443,#21444,
#21445,#21446,#21447,#21448,#21449,#21450),.UNSPECIFIED.,.F.,.F.,(4,1,1,
1,1,1,1,1,4),(47.1238898038469,47.3704174554844,48.3569467941484,49.3434761328125,
50.3300054714765,51.3165348101405,52.3030641488046,53.2895934874686,53.4070751110265),
 .UNSPECIFIED.);
#2027=B_SPLINE_CURVE_WITH_KNOTS('',3,(#21451,#21452,#21453,#21454,#21455,
#21456,#21457,#21458,#21459,#21460),.UNSPECIFIED.,.F.,.F.,(4,1,1,1,1,1,
1,4),(47.1238898038469,47.9403976415489,48.9269269802129,49.9134563188769,
50.899985657541,51.886514996205,52.873044334869,53.4070751110265),
 .UNSPECIFIED.);
#2028=B_SPLINE_CURVE_WITH_KNOTS('',3,(#21465,#21466,#21467,#21468,#21469,
#21470,#21471,#21472,#21473,#21474),.UNSPECIFIED.,.F.,.F.,(4,1,1,1,1,1,
1,4),(40.8407044966673,41.4512414235002,42.4377707621643,43.4243001008283,
44.4108294394923,45.3973587781563,46.3838881168204,47.1238898038469),
 .UNSPECIFIED.);
#2029=B_SPLINE_CURVE_WITH_KNOTS('',3,(#21475,#21476,#21477,#21478,#21479,
#21480,#21481,#21482,#21483,#21484,#21485),.UNSPECIFIED.,.F.,.F.,(4,1,1,
1,1,1,1,1,4),(40.8407044966673,41.0346922709007,42.0212216095647,43.0077509482287,
43.9942802868928,44.9808096255568,45.9673389642208,46.9538683028848,47.1238898038469),
 .UNSPECIFIED.);
#2030=B_SPLINE_CURVE_WITH_KNOTS('',3,(#21490,#21491,#21492,#21493,#21494,
#21495,#21496,#21497,#21498,#21499),.UNSPECIFIED.,.F.,.F.,(4,1,1,1,1,1,
1,4),(34.5575191894877,35.532065391516,36.5185947301801,37.5051240688441,
38.4916534075081,39.4781827461722,40.4647120848362,40.8407044966673),
 .UNSPECIFIED.);
#2031=B_SPLINE_CURVE_WITH_KNOTS('',3,(#21500,#21501,#21502,#21503,#21504,
#21505,#21506,#21507,#21508,#21509),.UNSPECIFIED.,.F.,.F.,(4,1,1,1,1,1,
1,4),(34.5575191894877,35.1155162389165,36.1020455775805,37.0885749162445,
38.0751042549086,39.0616335935726,40.0481629322366,40.8407044966673),
 .UNSPECIFIED.);
#2032=B_SPLINE_CURVE_WITH_KNOTS('',3,(#21514,#21515,#21516,#21517,#21518,
#21519,#21520,#21521,#21522,#21523,#21524),.UNSPECIFIED.,.F.,.F.,(4,1,1,
1,1,1,1,1,4),(28.2743338823081,28.6263600208678,29.6128893595319,30.5994186981959,
31.5859480368599,32.5724773755239,33.559006714188,34.545536052852,34.5575191894877),
 .UNSPECIFIED.);
#2033=B_SPLINE_CURVE_WITH_KNOTS('',3,(#21525,#21526,#21527,#21528,#21529,
#21530,#21531,#21532,#21533,#21534),.UNSPECIFIED.,.F.,.F.,(4,1,1,1,1,1,
1,4),(28.2743338823081,29.1963402069323,30.1828695455963,31.1693988842604,
32.1559282229244,33.1424575615884,34.1289869002524,34.5575191894877),
 .UNSPECIFIED.);
#2034=B_SPLINE_CURVE_WITH_KNOTS('',3,(#21539,#21540,#21541,#21542,#21543,
#21544,#21545,#21546,#21547,#21548),.UNSPECIFIED.,.F.,.F.,(4,1,1,1,1,1,
1,4),(21.9911485751285,22.7071839888836,23.6937133275477,24.6802426662117,
25.6667720048757,26.6533013435398,27.6398306822038,28.2743338823081),
 .UNSPECIFIED.);
#2035=B_SPLINE_CURVE_WITH_KNOTS('',3,(#21549,#21550,#21551,#21552,#21553,
#21554,#21555,#21556,#21557,#21558,#21559),.UNSPECIFIED.,.F.,.F.,(4,1,1,
1,1,1,1,1,4),(21.9911485751285,22.2906348362841,23.2771641749481,24.2636935136121,
25.2502228522762,26.2367521909402,27.2232815296042,28.2098108682683,28.2743338823081),
 .UNSPECIFIED.);
#2036=B_SPLINE_CURVE_WITH_KNOTS('',3,(#21565,#21566,#21567,#21568,#21569),
 .UNSPECIFIED.,.F.,.F.,(4,1,4),(14.3984001269718,15.3849294656359,15.707963267949),
 .UNSPECIFIED.);
#2037=B_SPLINE_CURVE_WITH_KNOTS('',3,(#21572,#21573,#21574,#21575,#21576),
 .UNSPECIFIED.,.F.,.F.,(4,1,4),(13.8759337553362,14.8149492795714,15.7079632679489),
 .UNSPECIFIED.);
#2038=B_SPLINE_CURVE_WITH_KNOTS('',3,(#21578,#21579,#21580,#21581,#21582,
#21583,#21584,#21585,#21586,#21587,#21588),.UNSPECIFIED.,.F.,.F.,(4,1,1,
1,1,1,1,1,4),(15.7079632679489,15.8014786182354,16.7880079568995,17.7745372955635,
18.7610666342275,19.7475959728915,20.7341253115556,21.7206546502196,21.9911485751285),
 .UNSPECIFIED.);
#2039=B_SPLINE_CURVE_WITH_KNOTS('',3,(#21589,#21590,#21591,#21592,#21593,
#21594,#21595,#21596,#21597,#21598),.UNSPECIFIED.,.F.,.F.,(4,1,1,1,1,1,
1,4),(15.707963267949,16.3714588042999,17.3579881429639,18.344517481628,
19.331046820292,20.317576158956,21.30410549762,21.9911485751285),
 .UNSPECIFIED.);
#2040=B_SPLINE_CURVE_WITH_KNOTS('',3,(#21823,#21824,#21825,#21826,#21827,
#21828,#21829,#21830,#21831,#21832,#21833,#21834,#21835,#21836,#21837,#21838,
#21839,#21840,#21841,#21842,#21843,#21844,#21845,#21846,#21847,#21848,#21849,
#21850,#21851,#21852,#21853,#21854,#21855,#21856,#21857,#21858,#21859,#21860,
#21861,#21862,#21863,#21864,#21865,#21866,#21867,#21868,#21869,#21870,#21871,
#21872,#21873,#21874),.UNSPECIFIED.,.F.,.F.,(4,3,3,3,3,3,3,3,3,3,3,3,3,
3,3,3,3,4),(0.,0.0320331684328983,0.047982254793735,0.0587463569853809,
0.068374331906695,0.0996455206564278,0.112637667143497,0.122453511831961,
0.146764141737192,0.169126652772842,0.178509832567225,0.203948034872107,
0.222826517887668,0.233934300135679,0.251364503567911,0.26339901807632,
0.280262641786753,0.286347380332264),.UNSPECIFIED.);
#2041=B_SPLINE_CURVE_WITH_KNOTS('',3,(#21875,#21876,#21877,#21878,#21879,
#21880,#21881,#21882,#21883,#21884,#21885,#21886,#21887,#21888,#21889,#21890,
#21891,#21892,#21893,#21894,#21895,#21896,#21897,#21898,#21899,#21900,#21901,
#21902,#21903,#21904,#21905,#21906,#21907,#21908,#21909,#21910,#21911,#21912,
#21913,#21914,#21915,#21916,#21917,#21918,#21919,#21920,#21921,#21922,#21923),
 .UNSPECIFIED.,.F.,.F.,(4,3,3,3,3,3,3,3,3,3,3,3,3,3,3,3,4),(0.,0.0274255978447832,
0.048809316595412,0.0580010326491972,0.0875347374149519,0.101224292480011,
0.111280556216297,0.132431451325231,0.155780476821444,0.165670961223459,
0.193708256295631,0.208717590629974,0.219760914288732,0.239138299607853,
0.257256761910142,0.277820141512149,0.28514280399518),.UNSPECIFIED.);
#2042=B_SPLINE_CURVE_WITH_KNOTS('',3,(#21924,#21925,#21926,#21927,#21928,
#21929,#21930,#21931,#21932,#21933,#21934,#21935,#21936,#21937,#21938,#21939,
#21940,#21941,#21942,#21943,#21944,#21945,#21946,#21947,#21948),
 .UNSPECIFIED.,.F.,.F.,(4,3,3,3,3,3,3,3,4),(-10.1357873115492,-9.8652933866403,
-8.87876404797627,-7.89223470931224,-6.90570537064821,-5.91917603198418,
-4.93264669332015,-3.94611735465612,-3.85260200436966),.UNSPECIFIED.);
#2043=B_SPLINE_CURVE_WITH_KNOTS('',3,(#22173,#22174,#22175,#22176,#22177,
#22178,#22179,#22180,#22181,#22182,#22183,#22184,#22185,#22186,#22187,#22188,
#22189,#22190,#22191,#22192,#22193,#22194,#22195,#22196,#22197,#22198,#22199,
#22200,#22201,#22202,#22203,#22204,#22205,#22206,#22207,#22208,#22209,#22210,
#22211,#22212,#22213,#22214,#22215,#22216,#22217,#22218,#22219,#22220,#22221),
 .UNSPECIFIED.,.F.,.F.,(4,3,3,3,3,3,3,3,3,3,3,3,3,3,3,3,4),(0.,0.0274255913653339,
0.0488093131133246,0.0580010269694127,0.0875347308595416,0.101224269152377,
0.111280553657591,0.132431451325227,0.155780477659062,0.165670961808075,
0.193708256734092,0.208717605217266,0.21976091765614,0.239138308570995,
0.257256762582239,0.277820141512144,0.28514280399514),.UNSPECIFIED.);
#2044=B_SPLINE_CURVE_WITH_KNOTS('',3,(#22222,#22223,#22224,#22225,#22226,
#22227,#22228,#22229,#22230,#22231,#22232,#22233,#22234,#22235,#22236,#22237,
#22238,#22239,#22240,#22241,#22242,#22243,#22244,#22245,#22246),
 .UNSPECIFIED.,.F.,.F.,(4,3,3,3,3,3,3,3,4),(7.5927484481567,7.89223470931224,
8.87876404797628,9.86529338664031,10.8518227253043,11.8383520639684,12.8248814026324,
13.8114107412964,13.8759337553363),.UNSPECIFIED.);
#2045=B_SPLINE_CURVE_WITH_KNOTS('',3,(#22247,#22248,#22249,#22250,#22251,
#22252,#22253,#22254,#22255,#22256,#22257,#22258,#22259,#22260,#22261,#22262,
#22263,#22264,#22265,#22266,#22267,#22268,#22269,#22270,#22271,#22272,#22273,
#22274,#22275,#22276,#22277,#22278,#22279,#22280,#22281,#22282,#22283,#22284,
#22285,#22286,#22287,#22288,#22289,#22290,#22291,#22292,#22293,#22294,#22295,
#22296,#22297,#22298),.UNSPECIFIED.,.F.,.F.,(4,3,3,3,3,3,3,3,3,3,3,3,3,
3,3,3,3,4),(0.,0.0320331645440323,0.0479822944538874,0.0587463983360561,
0.0683743388328265,0.0996455292883743,0.112637688108393,0.122453518454582,
0.146764141737195,0.169126651893336,0.178509831787203,0.20394803428708,
0.222826505940554,0.233934299906464,0.251364515046202,0.263399023832158,
0.280262641786714,0.28634738033223),.UNSPECIFIED.);
#2046=B_SPLINE_CURVE_WITH_KNOTS('',3,(#22312,#22313,#22314,#22315,#22316,
#22317,#22318,#22319,#22320,#22321,#22322,#22323,#22324,#22325,#22326,#22327,
#22328,#22329,#22330,#22331,#22332,#22333,#22334,#22335,#22336,#22337,#22338,
#22339,#22340,#22341,#22342,#22343,#22344,#22345,#22346,#22347,#22348,#22349,
#22350,#22351,#22352,#22353,#22354,#22355,#22356,#22357,#22358,#22359,#22360),
 .UNSPECIFIED.,.F.,.F.,(4,3,3,3,3,3,3,3,3,3,3,3,3,3,3,3,4),(0.,0.0274256070877454,
0.0488093215641943,0.0580010407627361,0.0875347467776894,0.101224325795315,
0.111280559869577,0.132431451325226,0.155780475624762,0.165670960389251,
0.193708255669975,0.208717569845021,0.219760909477782,0.239138286790648,
0.257256760954527,0.277820141512144,0.285142803995137),.UNSPECIFIED.);
#2047=B_SPLINE_CURVE_WITH_KNOTS('',3,(#22361,#22362,#22363,#22364,#22365,
#22366,#22367,#22368,#22369,#22370,#22371,#22372,#22373,#22374,#22375,#22376,
#22377,#22378,#22379,#22380,#22381,#22382,#22383,#22384,#22385,#22386,#22387,
#22388,#22389,#22390,#22391,#22392,#22393,#22394,#22395,#22396,#22397,#22398,
#22399,#22400,#22401,#22402,#22403,#22404,#22405,#22406,#22407,#22408,#22409,
#22410,#22411,#22412),.UNSPECIFIED.,.F.,.F.,(4,3,3,3,3,3,3,3,3,3,3,3,3,
3,3,3,3,4),(0.,0.032033144059138,0.0479825033685422,0.058746616231457,0.068374375333449,
0.0996455747709087,0.112637798572108,0.122453553351573,0.146764141737196,
0.169126647261903,0.17850982771232,0.203948031230928,0.22282644299279,0.233934298697096,
0.251364575521066,0.263399054117863,0.280262641786752,0.286347380332261),
 .UNSPECIFIED.);
#2048=B_SPLINE_CURVE_WITH_KNOTS('',3,(#22414,#22415,#22416,#22417,#22418,
#22419,#22420,#22421,#22422,#22423,#22424),.UNSPECIFIED.,.F.,.F.,(4,1,1,
1,1,1,1,1,4),(15.7079632679489,15.8014786182354,16.7880079568995,17.7745372955635,
18.7610666342275,19.7475959728915,20.7341253115556,21.7206546502196,21.9911485751285),
 .UNSPECIFIED.);
#2049=B_SPLINE_CURVE_WITH_KNOTS('',3,(#22425,#22426,#22427,#22428,#22429,
#22430,#22431,#22432,#22433,#22434),.UNSPECIFIED.,.F.,.F.,(4,1,1,1,1,1,
1,4),(15.707963267949,16.3714588042999,17.3579881429639,18.344517481628,
19.331046820292,20.317576158956,21.30410549762,21.9911485751285),
 .UNSPECIFIED.);
#2050=B_SPLINE_CURVE_WITH_KNOTS('',3,(#22659,#22660,#22661,#22662,#22663,
#22664,#22665,#22666,#22667,#22668,#22669,#22670,#22671,#22672,#22673,#22674,
#22675,#22676,#22677,#22678,#22679,#22680,#22681,#22682,#22683,#22684,#22685,
#22686,#22687,#22688,#22689,#22690,#22691,#22692,#22693,#22694,#22695,#22696,
#22697,#22698,#22699,#22700,#22701,#22702,#22703,#22704,#22705,#22706,#22707),
 .UNSPECIFIED.,.F.,.F.,(4,3,3,3,3,3,3,3,3,3,3,3,3,3,3,3,4),(0.,0.0274255572386018,
0.0488092947703195,0.0580009970300377,0.0875346963040298,0.101224146180659,
0.111280540172636,0.132431451325231,0.155780482071967,0.165670964883965,
0.19370825904101,0.208717681926172,0.219760935414438,0.239138355867989,
0.257256766122231,0.277820141512143,0.285142803995174),.UNSPECIFIED.);
#2051=B_SPLINE_CURVE_WITH_KNOTS('',3,(#22708,#22709,#22710,#22711,#22712,
#22713,#22714,#22715,#22716,#22717,#22718,#22719,#22720,#22721,#22722,#22723,
#22724,#22725,#22726,#22727,#22728,#22729,#22730,#22731,#22732),
 .UNSPECIFIED.,.F.,.F.,(4,3,3,3,3,3,3,3,4),(-10.1357873115492,-9.8652933866403,
-8.87876404797628,-7.89223470931224,-6.90570537064821,-5.91917603198418,
-4.93264669332015,-3.94611735465612,-3.85260200436966),.UNSPECIFIED.);
#2052=B_SPLINE_CURVE_WITH_KNOTS('',3,(#22957,#22958,#22959,#22960,#22961,
#22962,#22963,#22964,#22965,#22966,#22967,#22968,#22969,#22970,#22971,#22972,
#22973,#22974,#22975,#22976,#22977,#22978,#22979,#22980,#22981),
 .UNSPECIFIED.,.F.,.F.,(4,3,3,3,3,3,3,3,4),(7.5927484481567,7.89223470931225,
8.87876404797628,9.86529338664031,10.8518227253043,11.8383520639684,12.8248814026324,
13.8114107412964,13.8759337553363),.UNSPECIFIED.);
#2053=B_SPLINE_CURVE_WITH_KNOTS('',3,(#22982,#22983,#22984,#22985,#22986,
#22987,#22988,#22989,#22990,#22991,#22992,#22993,#22994,#22995,#22996,#22997,
#22998,#22999,#23000,#23001,#23002,#23003,#23004,#23005,#23006,#23007,#23008,
#23009,#23010,#23011,#23012,#23013,#23014,#23015,#23016,#23017,#23018,#23019,
#23020,#23021,#23022,#23023,#23024,#23025,#23026,#23027,#23028,#23029,#23030,
#23031,#23032,#23033),.UNSPECIFIED.,.F.,.F.,(4,3,3,3,3,3,3,3,3,3,3,3,3,
3,3,3,3,4),(0.,0.0320331739806594,0.047982198208099,0.0587462979950865,
0.0683743220264688,0.0996455083427913,0.112637637236076,0.122453502382791,
0.146764141737189,0.169126654027335,0.178509833663637,0.203948035694404,
0.222826534951851,0.233934300464251,0.251364487179106,0.263399009878289,
0.280262641786705,0.286347380332219),.UNSPECIFIED.);
#2630=LINE('',#20482,#3204);
#2631=LINE('',#20503,#3205);
#2632=LINE('',#20554,#3206);
#2633=LINE('',#20605,#3207);
#2634=LINE('',#20653,#3208);
#2635=LINE('',#20704,#3209);
#2636=LINE('',#20755,#3210);
#2637=LINE('',#20803,#3211);
#2638=LINE('',#20842,#3212);
#2639=LINE('',#20863,#3213);
#2640=LINE('',#20914,#3214);
#2641=LINE('',#20965,#3215);
#2642=LINE('',#21013,#3216);
#2643=LINE('',#21064,#3217);
#2644=LINE('',#21115,#3218);
#2645=LINE('',#21163,#3219);
#2646=LINE('',#21202,#3220);
#2647=LINE('',#21226,#3221);
#2648=LINE('',#21250,#3222);
#2649=LINE('',#21275,#3223);
#2650=LINE('',#21300,#3224);
#2651=LINE('',#21324,#3225);
#2652=LINE('',#21349,#3226);
#2653=LINE('',#21374,#3227);
#2654=LINE('',#21391,#3228);
#2655=LINE('',#21415,#3229);
#2656=LINE('',#21439,#3230);
#2657=LINE('',#21464,#3231);
#2658=LINE('',#21489,#3232);
#2659=LINE('',#21513,#3233);
#2660=LINE('',#21538,#3234);
#2661=LINE('',#21563,#3235);
#2662=LINE('',#22304,#3236);
#2663=LINE('',#22306,#3237);
#2664=LINE('',#22308,#3238);
#2665=LINE('',#22310,#3239);
#2666=LINE('',#22311,#3240);
#2667=LINE('',#23040,#3241);
#2668=LINE('',#23046,#3242);
#2669=LINE('',#23051,#3243);
#2670=LINE('',#23053,#3244);
#2671=LINE('',#23055,#3245);
#2672=LINE('',#23056,#3246);
#2673=LINE('',#23059,#3247);
#2674=LINE('',#23061,#3248);
#2675=LINE('',#23062,#3249);
#2676=LINE('',#23065,#3250);
#2677=LINE('',#23067,#3251);
#2678=LINE('',#23069,#3252);
#2679=LINE('',#23071,#3253);
#2680=LINE('',#23073,#3254);
#2681=LINE('',#23075,#3255);
#2682=LINE('',#23076,#3256);
#2683=LINE('',#23079,#3257);
#2684=LINE('',#23080,#3258);
#2685=LINE('',#23083,#3259);
#2686=LINE('',#23084,#3260);
#2687=LINE('',#23087,#3261);
#2688=LINE('',#23088,#3262);
#2689=LINE('',#23093,#3263);
#2690=LINE('',#23094,#3264);
#2691=LINE('',#23099,#3265);
#2692=LINE('',#23100,#3266);
#2693=LINE('',#23103,#3267);
#2694=LINE('',#23104,#3268);
#2695=LINE('',#23109,#3269);
#2696=LINE('',#23111,#3270);
#2697=LINE('',#23112,#3271);
#2698=LINE('',#23115,#3272);
#2699=LINE('',#23117,#3273);
#2700=LINE('',#23118,#3274);
#2701=LINE('',#23120,#3275);
#2702=LINE('',#23123,#3276);
#2703=LINE('',#23125,#3277);
#2704=LINE('',#23126,#3278);
#2705=LINE('',#23128,#3279);
#2706=LINE('',#23133,#3280);
#3204=VECTOR('',#11349,0.15);
#3205=VECTOR('',#11354,0.15);
#3206=VECTOR('',#11357,0.15);
#3207=VECTOR('',#11360,0.15);
#3208=VECTOR('',#11363,0.15);
#3209=VECTOR('',#11366,0.15);
#3210=VECTOR('',#11369,0.15);
#3211=VECTOR('',#11372,0.15);
#3212=VECTOR('',#11377,0.15);
#3213=VECTOR('',#11382,0.15);
#3214=VECTOR('',#11385,0.15);
#3215=VECTOR('',#11388,0.15);
#3216=VECTOR('',#11391,0.15);
#3217=VECTOR('',#11394,0.15);
#3218=VECTOR('',#11397,0.15);
#3219=VECTOR('',#11400,0.15);
#3220=VECTOR('',#11405,0.1543);
#3221=VECTOR('',#11410,0.1543);
#3222=VECTOR('',#11413,0.1543);
#3223=VECTOR('',#11416,0.1543);
#3224=VECTOR('',#11419,0.1543);
#3225=VECTOR('',#11422,0.1543);
#3226=VECTOR('',#11425,0.1543);
#3227=VECTOR('',#11428,0.1543);
#3228=VECTOR('',#11433,0.1543);
#3229=VECTOR('',#11438,0.1543);
#3230=VECTOR('',#11441,0.1543);
#3231=VECTOR('',#11444,0.1543);
#3232=VECTOR('',#11447,0.1543);
#3233=VECTOR('',#11450,0.1543);
#3234=VECTOR('',#11453,0.1543);
#3235=VECTOR('',#11456,0.1543);
#3236=VECTOR('',#11465,1.);
#3237=VECTOR('',#11466,1.);
#3238=VECTOR('',#11467,1.);
#3239=VECTOR('',#11468,1.);
#3240=VECTOR('',#11469,1.);
#3241=VECTOR('',#11480,0.2);
#3242=VECTOR('',#11487,0.2);
#3243=VECTOR('',#11492,1.);
#3244=VECTOR('',#11493,1.);
#3245=VECTOR('',#11494,1.);
#3246=VECTOR('',#11495,1.);
#3247=VECTOR('',#11498,1.);
#3248=VECTOR('',#11499,1.);
#3249=VECTOR('',#11500,1.);
#3250=VECTOR('',#11503,1.);
#3251=VECTOR('',#11504,1.);
#3252=VECTOR('',#11505,1.);
#3253=VECTOR('',#11506,1.);
#3254=VECTOR('',#11507,1.);
#3255=VECTOR('',#11508,1.);
#3256=VECTOR('',#11509,1.);
#3257=VECTOR('',#11512,1.);
#3258=VECTOR('',#11513,1.);
#3259=VECTOR('',#11516,1.);
#3260=VECTOR('',#11517,1.);
#3261=VECTOR('',#11520,1.);
#3262=VECTOR('',#11521,1.);
#3263=VECTOR('',#11526,1.);
#3264=VECTOR('',#11527,1.);
#3265=VECTOR('',#11532,1.);
#3266=VECTOR('',#11533,1.);
#3267=VECTOR('',#11538,1.);
#3268=VECTOR('',#11539,1.);
#3269=VECTOR('',#11546,1.);
#3270=VECTOR('',#11547,1.);
#3271=VECTOR('',#11548,1.);
#3272=VECTOR('',#11551,1.);
#3273=VECTOR('',#11552,1.);
#3274=VECTOR('',#11553,1.);
#3275=VECTOR('',#11556,1.);
#3276=VECTOR('',#11559,1.);
#3277=VECTOR('',#11560,1.);
#3278=VECTOR('',#11561,1.);
#3279=VECTOR('',#11564,1.);
#3280=VECTOR('',#11571,0.6);
#3915=VERTEX_POINT('',#20480);
#3916=VERTEX_POINT('',#20481);
#3917=VERTEX_POINT('',#20483);
#3918=VERTEX_POINT('',#20488);
#3919=VERTEX_POINT('',#20501);
#3920=VERTEX_POINT('',#20502);
#3921=VERTEX_POINT('',#20552);
#3922=VERTEX_POINT('',#20553);
#3923=VERTEX_POINT('',#20603);
#3924=VERTEX_POINT('',#20604);
#3925=VERTEX_POINT('',#20651);
#3926=VERTEX_POINT('',#20652);
#3927=VERTEX_POINT('',#20702);
#3928=VERTEX_POINT('',#20703);
#3929=VERTEX_POINT('',#20753);
#3930=VERTEX_POINT('',#20754);
#3931=VERTEX_POINT('',#20801);
#3932=VERTEX_POINT('',#20802);
#3933=VERTEX_POINT('',#20804);
#3934=VERTEX_POINT('',#20818);
#3935=VERTEX_POINT('',#20840);
#3936=VERTEX_POINT('',#20841);
#3937=VERTEX_POINT('',#20843);
#3938=VERTEX_POINT('',#20848);
#3939=VERTEX_POINT('',#20861);
#3940=VERTEX_POINT('',#20862);
#3941=VERTEX_POINT('',#20912);
#3942=VERTEX_POINT('',#20913);
#3943=VERTEX_POINT('',#20963);
#3944=VERTEX_POINT('',#20964);
#3945=VERTEX_POINT('',#21011);
#3946=VERTEX_POINT('',#21012);
#3947=VERTEX_POINT('',#21062);
#3948=VERTEX_POINT('',#21063);
#3949=VERTEX_POINT('',#21113);
#3950=VERTEX_POINT('',#21114);
#3951=VERTEX_POINT('',#21161);
#3952=VERTEX_POINT('',#21162);
#3953=VERTEX_POINT('',#21164);
#3954=VERTEX_POINT('',#21178);
#3955=VERTEX_POINT('',#21200);
#3956=VERTEX_POINT('',#21201);
#3957=VERTEX_POINT('',#21203);
#3958=VERTEX_POINT('',#21212);
#3959=VERTEX_POINT('',#21224);
#3960=VERTEX_POINT('',#21225);
#3961=VERTEX_POINT('',#21248);
#3962=VERTEX_POINT('',#21249);
#3963=VERTEX_POINT('',#21273);
#3964=VERTEX_POINT('',#21274);
#3965=VERTEX_POINT('',#21298);
#3966=VERTEX_POINT('',#21299);
#3967=VERTEX_POINT('',#21322);
#3968=VERTEX_POINT('',#21323);
#3969=VERTEX_POINT('',#21347);
#3970=VERTEX_POINT('',#21348);
#3971=VERTEX_POINT('',#21372);
#3972=VERTEX_POINT('',#21373);
#3973=VERTEX_POINT('',#21375);
#3974=VERTEX_POINT('',#21381);
#3975=VERTEX_POINT('',#21389);
#3976=VERTEX_POINT('',#21390);
#3977=VERTEX_POINT('',#21392);
#3978=VERTEX_POINT('',#21401);
#3979=VERTEX_POINT('',#21413);
#3980=VERTEX_POINT('',#21414);
#3981=VERTEX_POINT('',#21437);
#3982=VERTEX_POINT('',#21438);
#3983=VERTEX_POINT('',#21462);
#3984=VERTEX_POINT('',#21463);
#3985=VERTEX_POINT('',#21487);
#3986=VERTEX_POINT('',#21488);
#3987=VERTEX_POINT('',#21511);
#3988=VERTEX_POINT('',#21512);
#3989=VERTEX_POINT('',#21536);
#3990=VERTEX_POINT('',#21537);
#3991=VERTEX_POINT('',#21561);
#3992=VERTEX_POINT('',#21562);
#3993=VERTEX_POINT('',#21564);
#3994=VERTEX_POINT('',#21570);
#3995=VERTEX_POINT('',#22300);
#3996=VERTEX_POINT('',#22301);
#3997=VERTEX_POINT('',#22303);
#3998=VERTEX_POINT('',#22305);
#3999=VERTEX_POINT('',#22307);
#4000=VERTEX_POINT('',#22309);
#4001=VERTEX_POINT('',#23037);
#4002=VERTEX_POINT('',#23039);
#4003=VERTEX_POINT('',#23043);
#4004=VERTEX_POINT('',#23045);
#4005=VERTEX_POINT('',#23049);
#4006=VERTEX_POINT('',#23050);
#4007=VERTEX_POINT('',#23052);
#4008=VERTEX_POINT('',#23054);
#4009=VERTEX_POINT('',#23058);
#4010=VERTEX_POINT('',#23060);
#4011=VERTEX_POINT('',#23064);
#4012=VERTEX_POINT('',#23066);
#4013=VERTEX_POINT('',#23068);
#4014=VERTEX_POINT('',#23070);
#4015=VERTEX_POINT('',#23072);
#4016=VERTEX_POINT('',#23074);
#4017=VERTEX_POINT('',#23078);
#4018=VERTEX_POINT('',#23082);
#4019=VERTEX_POINT('',#23086);
#4020=VERTEX_POINT('',#23090);
#4021=VERTEX_POINT('',#23092);
#4022=VERTEX_POINT('',#23096);
#4023=VERTEX_POINT('',#23098);
#4024=VERTEX_POINT('',#23108);
#4025=VERTEX_POINT('',#23110);
#4026=VERTEX_POINT('',#23114);
#4027=VERTEX_POINT('',#23116);
#4028=VERTEX_POINT('',#23122);
#4029=VERTEX_POINT('',#23124);
#4030=VERTEX_POINT('',#23132);
#5032=EDGE_CURVE('',#3915,#3916,#2630,.T.);
#5033=EDGE_CURVE('',#3916,#3917,#1974,.T.);
#5034=EDGE_CURVE('',#3918,#3917,#1644,.F.);
#5035=EDGE_CURVE('',#3918,#3915,#1975,.T.);
#5036=EDGE_CURVE('',#3919,#3920,#2631,.T.);
#5037=EDGE_CURVE('',#3920,#3916,#1976,.T.);
#5038=EDGE_CURVE('',#3915,#3919,#1977,.T.);
#5039=EDGE_CURVE('',#3921,#3922,#2632,.T.);
#5040=EDGE_CURVE('',#3922,#3920,#1978,.T.);
#5041=EDGE_CURVE('',#3919,#3921,#1979,.T.);
#5042=EDGE_CURVE('',#3923,#3924,#2633,.T.);
#5043=EDGE_CURVE('',#3924,#3922,#1980,.T.);
#5044=EDGE_CURVE('',#3921,#3923,#1981,.T.);
#5045=EDGE_CURVE('',#3925,#3926,#2634,.T.);
#5046=EDGE_CURVE('',#3926,#3924,#1982,.T.);
#5047=EDGE_CURVE('',#3923,#3925,#1983,.T.);
#5048=EDGE_CURVE('',#3927,#3928,#2635,.T.);
#5049=EDGE_CURVE('',#3928,#3926,#1984,.T.);
#5050=EDGE_CURVE('',#3925,#3927,#1985,.T.);
#5051=EDGE_CURVE('',#3929,#3930,#2636,.T.);
#5052=EDGE_CURVE('',#3930,#3928,#1986,.T.);
#5053=EDGE_CURVE('',#3927,#3929,#1987,.T.);
#5054=EDGE_CURVE('',#3931,#3932,#2637,.T.);
#5055=EDGE_CURVE('',#3931,#3933,#1988,.T.);
#5056=EDGE_CURVE('',#3934,#3933,#1645,.T.);
#5057=EDGE_CURVE('',#3934,#3932,#1989,.T.);
#5058=EDGE_CURVE('',#3935,#3936,#2638,.T.);
#5059=EDGE_CURVE('',#3936,#3937,#1990,.T.);
#5060=EDGE_CURVE('',#3938,#3937,#1646,.F.);
#5061=EDGE_CURVE('',#3938,#3935,#1991,.T.);
#5062=EDGE_CURVE('',#3939,#3940,#2639,.T.);
#5063=EDGE_CURVE('',#3940,#3936,#1992,.T.);
#5064=EDGE_CURVE('',#3935,#3939,#1993,.T.);
#5065=EDGE_CURVE('',#3941,#3942,#2640,.T.);
#5066=EDGE_CURVE('',#3942,#3940,#1994,.T.);
#5067=EDGE_CURVE('',#3939,#3941,#1995,.T.);
#5068=EDGE_CURVE('',#3943,#3944,#2641,.T.);
#5069=EDGE_CURVE('',#3944,#3942,#1996,.T.);
#5070=EDGE_CURVE('',#3941,#3943,#1997,.T.);
#5071=EDGE_CURVE('',#3945,#3946,#2642,.T.);
#5072=EDGE_CURVE('',#3946,#3944,#1998,.T.);
#5073=EDGE_CURVE('',#3943,#3945,#1999,.T.);
#5074=EDGE_CURVE('',#3947,#3948,#2643,.T.);
#5075=EDGE_CURVE('',#3948,#3946,#2000,.T.);
#5076=EDGE_CURVE('',#3945,#3947,#2001,.T.);
#5077=EDGE_CURVE('',#3949,#3950,#2644,.T.);
#5078=EDGE_CURVE('',#3950,#3948,#2002,.T.);
#5079=EDGE_CURVE('',#3947,#3949,#2003,.T.);
#5080=EDGE_CURVE('',#3951,#3952,#2645,.T.);
#5081=EDGE_CURVE('',#3951,#3953,#2004,.T.);
#5082=EDGE_CURVE('',#3954,#3953,#1647,.T.);
#5083=EDGE_CURVE('',#3954,#3952,#2005,.T.);
#5084=EDGE_CURVE('',#3955,#3956,#2646,.T.);
#5085=EDGE_CURVE('',#3956,#3957,#2006,.T.);
#5086=EDGE_CURVE('',#3958,#3957,#1648,.T.);
#5087=EDGE_CURVE('',#3955,#3958,#2007,.T.);
#5088=EDGE_CURVE('',#3959,#3960,#2647,.T.);
#5089=EDGE_CURVE('',#3960,#3956,#2008,.T.);
#5090=EDGE_CURVE('',#3959,#3955,#2009,.T.);
#5091=EDGE_CURVE('',#3961,#3962,#2648,.T.);
#5092=EDGE_CURVE('',#3962,#3960,#2010,.T.);
#5093=EDGE_CURVE('',#3961,#3959,#2011,.T.);
#5094=EDGE_CURVE('',#3963,#3964,#2649,.T.);
#5095=EDGE_CURVE('',#3964,#3962,#2012,.T.);
#5096=EDGE_CURVE('',#3963,#3961,#2013,.T.);
#5097=EDGE_CURVE('',#3965,#3966,#2650,.T.);
#5098=EDGE_CURVE('',#3966,#3964,#2014,.T.);
#5099=EDGE_CURVE('',#3965,#3963,#2015,.T.);
#5100=EDGE_CURVE('',#3967,#3968,#2651,.T.);
#5101=EDGE_CURVE('',#3968,#3966,#2016,.T.);
#5102=EDGE_CURVE('',#3967,#3965,#2017,.T.);
#5103=EDGE_CURVE('',#3969,#3970,#2652,.T.);
#5104=EDGE_CURVE('',#3970,#3968,#2018,.T.);
#5105=EDGE_CURVE('',#3969,#3967,#2019,.T.);
#5106=EDGE_CURVE('',#3971,#3972,#2653,.T.);
#5107=EDGE_CURVE('',#3973,#3971,#2020,.T.);
#5108=EDGE_CURVE('',#3974,#3973,#1649,.T.);
#5109=EDGE_CURVE('',#3974,#3972,#2021,.T.);
#5110=EDGE_CURVE('',#3975,#3976,#2654,.T.);
#5111=EDGE_CURVE('',#3976,#3977,#2022,.T.);
#5112=EDGE_CURVE('',#3978,#3977,#1650,.T.);
#5113=EDGE_CURVE('',#3975,#3978,#2023,.T.);
#5114=EDGE_CURVE('',#3979,#3980,#2655,.T.);
#5115=EDGE_CURVE('',#3980,#3976,#2024,.T.);
#5116=EDGE_CURVE('',#3979,#3975,#2025,.T.);
#5117=EDGE_CURVE('',#3981,#3982,#2656,.T.);
#5118=EDGE_CURVE('',#3982,#3980,#2026,.T.);
#5119=EDGE_CURVE('',#3981,#3979,#2027,.T.);
#5120=EDGE_CURVE('',#3983,#3984,#2657,.T.);
#5121=EDGE_CURVE('',#3984,#3982,#2028,.T.);
#5122=EDGE_CURVE('',#3983,#3981,#2029,.T.);
#5123=EDGE_CURVE('',#3985,#3986,#2658,.T.);
#5124=EDGE_CURVE('',#3986,#3984,#2030,.T.);
#5125=EDGE_CURVE('',#3985,#3983,#2031,.T.);
#5126=EDGE_CURVE('',#3987,#3988,#2659,.T.);
#5127=EDGE_CURVE('',#3988,#3986,#2032,.T.);
#5128=EDGE_CURVE('',#3987,#3985,#2033,.T.);
#5129=EDGE_CURVE('',#3989,#3990,#2660,.T.);
#5130=EDGE_CURVE('',#3990,#3988,#2034,.T.);
#5131=EDGE_CURVE('',#3989,#3987,#2035,.T.);
#5132=EDGE_CURVE('',#3991,#3992,#2661,.T.);
#5133=EDGE_CURVE('',#3993,#3991,#2036,.T.);
#5134=EDGE_CURVE('',#3994,#3993,#1651,.T.);
#5135=EDGE_CURVE('',#3994,#3992,#2037,.T.);
#5136=EDGE_CURVE('',#3992,#3990,#2038,.T.);
#5137=EDGE_CURVE('',#3991,#3989,#2039,.T.);
#5138=EDGE_CURVE('',#3977,#3938,#2040,.T.);
#5139=EDGE_CURVE('',#3953,#3994,#2041,.T.);
#5140=EDGE_CURVE('',#3949,#3951,#2042,.T.);
#5141=EDGE_CURVE('',#3937,#3978,#2043,.T.);
#5142=EDGE_CURVE('',#3952,#3950,#2044,.T.);
#5143=EDGE_CURVE('',#3993,#3954,#2045,.T.);
#5144=EDGE_CURVE('',#3995,#3996,#1652,.T.);
#5145=EDGE_CURVE('',#3997,#3995,#2662,.T.);
#5146=EDGE_CURVE('',#3998,#3997,#2663,.T.);
#5147=EDGE_CURVE('',#3999,#3998,#2664,.T.);
#5148=EDGE_CURVE('',#4000,#3999,#2665,.T.);
#5149=EDGE_CURVE('',#3996,#4000,#2666,.T.);
#5150=EDGE_CURVE('',#3917,#3958,#2046,.T.);
#5151=EDGE_CURVE('',#3957,#3918,#2047,.T.);
#5152=EDGE_CURVE('',#3972,#3970,#2048,.T.);
#5153=EDGE_CURVE('',#3971,#3969,#2049,.T.);
#5154=EDGE_CURVE('',#3933,#3974,#2050,.T.);
#5155=EDGE_CURVE('',#3929,#3931,#2051,.T.);
#5156=EDGE_CURVE('',#3932,#3930,#2052,.T.);
#5157=EDGE_CURVE('',#3973,#3934,#2053,.T.);
#5158=EDGE_CURVE('',#4001,#4001,#1653,.T.);
#5159=EDGE_CURVE('',#4001,#4002,#2667,.T.);
#5160=EDGE_CURVE('',#4002,#4002,#1654,.T.);
#5161=EDGE_CURVE('',#4003,#4003,#1655,.T.);
#5162=EDGE_CURVE('',#4003,#4004,#2668,.T.);
#5163=EDGE_CURVE('',#4004,#4004,#1656,.T.);
#5164=EDGE_CURVE('',#4005,#4006,#2669,.T.);
#5165=EDGE_CURVE('',#4005,#4007,#2670,.T.);
#5166=EDGE_CURVE('',#4008,#4007,#2671,.T.);
#5167=EDGE_CURVE('',#4006,#4008,#2672,.T.);
#5168=EDGE_CURVE('',#4007,#4009,#2673,.T.);
#5169=EDGE_CURVE('',#4009,#4010,#2674,.T.);
#5170=EDGE_CURVE('',#4010,#4008,#2675,.T.);
#5171=EDGE_CURVE('',#4011,#4009,#2676,.T.);
#5172=EDGE_CURVE('',#4012,#4005,#2677,.T.);
#5173=EDGE_CURVE('',#4012,#4013,#2678,.T.);
#5174=EDGE_CURVE('',#4014,#4013,#2679,.T.);
#5175=EDGE_CURVE('',#4015,#4014,#2680,.T.);
#5176=EDGE_CURVE('',#4015,#4016,#2681,.T.);
#5177=EDGE_CURVE('',#4016,#4011,#2682,.T.);
#5178=EDGE_CURVE('',#4006,#4017,#2683,.T.);
#5179=EDGE_CURVE('',#4017,#4012,#2684,.T.);
#5180=EDGE_CURVE('',#4017,#4018,#2685,.T.);
#5181=EDGE_CURVE('',#4013,#4018,#2686,.T.);
#5182=EDGE_CURVE('',#4019,#4014,#2687,.T.);
#5183=EDGE_CURVE('',#4018,#4019,#2688,.T.);
#5184=EDGE_CURVE('',#4020,#4016,#1657,.T.);
#5185=EDGE_CURVE('',#4021,#4020,#2689,.T.);
#5186=EDGE_CURVE('',#4011,#4021,#2690,.T.);
#5187=EDGE_CURVE('',#4016,#4022,#1658,.T.);
#5188=EDGE_CURVE('',#4023,#4015,#2691,.T.);
#5189=EDGE_CURVE('',#4020,#4023,#2692,.T.);
#5190=EDGE_CURVE('',#4022,#4020,#1659,.T.);
#5191=EDGE_CURVE('',#4021,#4010,#2693,.T.);
#5192=EDGE_CURVE('',#4023,#4019,#2694,.T.);
#5193=EDGE_CURVE('',#3996,#4024,#2695,.T.);
#5194=EDGE_CURVE('',#4000,#4025,#2696,.T.);
#5195=EDGE_CURVE('',#4024,#4025,#2697,.T.);
#5196=EDGE_CURVE('',#3998,#4026,#2698,.T.);
#5197=EDGE_CURVE('',#4027,#4026,#2699,.T.);
#5198=EDGE_CURVE('',#3999,#4027,#2700,.T.);
#5199=EDGE_CURVE('',#4025,#4027,#2701,.T.);
#5200=EDGE_CURVE('',#4028,#3995,#2702,.T.);
#5201=EDGE_CURVE('',#4029,#4028,#2703,.T.);
#5202=EDGE_CURVE('',#3997,#4029,#2704,.T.);
#5203=EDGE_CURVE('',#4026,#4029,#2705,.T.);
#5204=EDGE_CURVE('',#4028,#4024,#1660,.T.);
#5205=EDGE_CURVE('',#4022,#4030,#2706,.T.);
#5206=EDGE_CURVE('',#4030,#4030,#1661,.T.);
#6952=ORIENTED_EDGE('',*,*,#5032,.T.);
#6953=ORIENTED_EDGE('',*,*,#5033,.T.);
#6954=ORIENTED_EDGE('',*,*,#5034,.F.);
#6955=ORIENTED_EDGE('',*,*,#5035,.T.);
#6956=ORIENTED_EDGE('',*,*,#5036,.T.);
#6957=ORIENTED_EDGE('',*,*,#5037,.T.);
#6958=ORIENTED_EDGE('',*,*,#5032,.F.);
#6959=ORIENTED_EDGE('',*,*,#5038,.T.);
#6960=ORIENTED_EDGE('',*,*,#5039,.T.);
#6961=ORIENTED_EDGE('',*,*,#5040,.T.);
#6962=ORIENTED_EDGE('',*,*,#5036,.F.);
#6963=ORIENTED_EDGE('',*,*,#5041,.T.);
#6964=ORIENTED_EDGE('',*,*,#5042,.T.);
#6965=ORIENTED_EDGE('',*,*,#5043,.T.);
#6966=ORIENTED_EDGE('',*,*,#5039,.F.);
#6967=ORIENTED_EDGE('',*,*,#5044,.T.);
#6968=ORIENTED_EDGE('',*,*,#5045,.T.);
#6969=ORIENTED_EDGE('',*,*,#5046,.T.);
#6970=ORIENTED_EDGE('',*,*,#5042,.F.);
#6971=ORIENTED_EDGE('',*,*,#5047,.T.);
#6972=ORIENTED_EDGE('',*,*,#5048,.T.);
#6973=ORIENTED_EDGE('',*,*,#5049,.T.);
#6974=ORIENTED_EDGE('',*,*,#5045,.F.);
#6975=ORIENTED_EDGE('',*,*,#5050,.T.);
#6976=ORIENTED_EDGE('',*,*,#5051,.T.);
#6977=ORIENTED_EDGE('',*,*,#5052,.T.);
#6978=ORIENTED_EDGE('',*,*,#5048,.F.);
#6979=ORIENTED_EDGE('',*,*,#5053,.T.);
#6980=ORIENTED_EDGE('',*,*,#5054,.F.);
#6981=ORIENTED_EDGE('',*,*,#5055,.T.);
#6982=ORIENTED_EDGE('',*,*,#5056,.F.);
#6983=ORIENTED_EDGE('',*,*,#5057,.T.);
#6984=ORIENTED_EDGE('',*,*,#5058,.T.);
#6985=ORIENTED_EDGE('',*,*,#5059,.T.);
#6986=ORIENTED_EDGE('',*,*,#5060,.F.);
#6987=ORIENTED_EDGE('',*,*,#5061,.T.);
#6988=ORIENTED_EDGE('',*,*,#5062,.T.);
#6989=ORIENTED_EDGE('',*,*,#5063,.T.);
#6990=ORIENTED_EDGE('',*,*,#5058,.F.);
#6991=ORIENTED_EDGE('',*,*,#5064,.T.);
#6992=ORIENTED_EDGE('',*,*,#5065,.T.);
#6993=ORIENTED_EDGE('',*,*,#5066,.T.);
#6994=ORIENTED_EDGE('',*,*,#5062,.F.);
#6995=ORIENTED_EDGE('',*,*,#5067,.T.);
#6996=ORIENTED_EDGE('',*,*,#5068,.T.);
#6997=ORIENTED_EDGE('',*,*,#5069,.T.);
#6998=ORIENTED_EDGE('',*,*,#5065,.F.);
#6999=ORIENTED_EDGE('',*,*,#5070,.T.);
#7000=ORIENTED_EDGE('',*,*,#5071,.T.);
#7001=ORIENTED_EDGE('',*,*,#5072,.T.);
#7002=ORIENTED_EDGE('',*,*,#5068,.F.);
#7003=ORIENTED_EDGE('',*,*,#5073,.T.);
#7004=ORIENTED_EDGE('',*,*,#5074,.T.);
#7005=ORIENTED_EDGE('',*,*,#5075,.T.);
#7006=ORIENTED_EDGE('',*,*,#5071,.F.);
#7007=ORIENTED_EDGE('',*,*,#5076,.T.);
#7008=ORIENTED_EDGE('',*,*,#5077,.T.);
#7009=ORIENTED_EDGE('',*,*,#5078,.T.);
#7010=ORIENTED_EDGE('',*,*,#5074,.F.);
#7011=ORIENTED_EDGE('',*,*,#5079,.T.);
#7012=ORIENTED_EDGE('',*,*,#5080,.F.);
#7013=ORIENTED_EDGE('',*,*,#5081,.T.);
#7014=ORIENTED_EDGE('',*,*,#5082,.F.);
#7015=ORIENTED_EDGE('',*,*,#5083,.T.);
#7016=ORIENTED_EDGE('',*,*,#5084,.T.);
#7017=ORIENTED_EDGE('',*,*,#5085,.T.);
#7018=ORIENTED_EDGE('',*,*,#5086,.F.);
#7019=ORIENTED_EDGE('',*,*,#5087,.F.);
#7020=ORIENTED_EDGE('',*,*,#5088,.T.);
#7021=ORIENTED_EDGE('',*,*,#5089,.T.);
#7022=ORIENTED_EDGE('',*,*,#5084,.F.);
#7023=ORIENTED_EDGE('',*,*,#5090,.F.);
#7024=ORIENTED_EDGE('',*,*,#5091,.T.);
#7025=ORIENTED_EDGE('',*,*,#5092,.T.);
#7026=ORIENTED_EDGE('',*,*,#5088,.F.);
#7027=ORIENTED_EDGE('',*,*,#5093,.F.);
#7028=ORIENTED_EDGE('',*,*,#5094,.T.);
#7029=ORIENTED_EDGE('',*,*,#5095,.T.);
#7030=ORIENTED_EDGE('',*,*,#5091,.F.);
#7031=ORIENTED_EDGE('',*,*,#5096,.F.);
#7032=ORIENTED_EDGE('',*,*,#5097,.T.);
#7033=ORIENTED_EDGE('',*,*,#5098,.T.);
#7034=ORIENTED_EDGE('',*,*,#5094,.F.);
#7035=ORIENTED_EDGE('',*,*,#5099,.F.);
#7036=ORIENTED_EDGE('',*,*,#5100,.T.);
#7037=ORIENTED_EDGE('',*,*,#5101,.T.);
#7038=ORIENTED_EDGE('',*,*,#5097,.F.);
#7039=ORIENTED_EDGE('',*,*,#5102,.F.);
#7040=ORIENTED_EDGE('',*,*,#5103,.T.);
#7041=ORIENTED_EDGE('',*,*,#5104,.T.);
#7042=ORIENTED_EDGE('',*,*,#5100,.F.);
#7043=ORIENTED_EDGE('',*,*,#5105,.F.);
#7044=ORIENTED_EDGE('',*,*,#5106,.F.);
#7045=ORIENTED_EDGE('',*,*,#5107,.F.);
#7046=ORIENTED_EDGE('',*,*,#5108,.F.);
#7047=ORIENTED_EDGE('',*,*,#5109,.T.);
#7048=ORIENTED_EDGE('',*,*,#5110,.T.);
#7049=ORIENTED_EDGE('',*,*,#5111,.T.);
#7050=ORIENTED_EDGE('',*,*,#5112,.F.);
#7051=ORIENTED_EDGE('',*,*,#5113,.F.);
#7052=ORIENTED_EDGE('',*,*,#5114,.T.);
#7053=ORIENTED_EDGE('',*,*,#5115,.T.);
#7054=ORIENTED_EDGE('',*,*,#5110,.F.);
#7055=ORIENTED_EDGE('',*,*,#5116,.F.);
#7056=ORIENTED_EDGE('',*,*,#5117,.T.);
#7057=ORIENTED_EDGE('',*,*,#5118,.T.);
#7058=ORIENTED_EDGE('',*,*,#5114,.F.);
#7059=ORIENTED_EDGE('',*,*,#5119,.F.);
#7060=ORIENTED_EDGE('',*,*,#5120,.T.);
#7061=ORIENTED_EDGE('',*,*,#5121,.T.);
#7062=ORIENTED_EDGE('',*,*,#5117,.F.);
#7063=ORIENTED_EDGE('',*,*,#5122,.F.);
#7064=ORIENTED_EDGE('',*,*,#5123,.T.);
#7065=ORIENTED_EDGE('',*,*,#5124,.T.);
#7066=ORIENTED_EDGE('',*,*,#5120,.F.);
#7067=ORIENTED_EDGE('',*,*,#5125,.F.);
#7068=ORIENTED_EDGE('',*,*,#5126,.T.);
#7069=ORIENTED_EDGE('',*,*,#5127,.T.);
#7070=ORIENTED_EDGE('',*,*,#5123,.F.);
#7071=ORIENTED_EDGE('',*,*,#5128,.F.);
#7072=ORIENTED_EDGE('',*,*,#5129,.T.);
#7073=ORIENTED_EDGE('',*,*,#5130,.T.);
#7074=ORIENTED_EDGE('',*,*,#5126,.F.);
#7075=ORIENTED_EDGE('',*,*,#5131,.F.);
#7076=ORIENTED_EDGE('',*,*,#5132,.F.);
#7077=ORIENTED_EDGE('',*,*,#5133,.F.);
#7078=ORIENTED_EDGE('',*,*,#5134,.F.);
#7079=ORIENTED_EDGE('',*,*,#5135,.T.);
#7080=ORIENTED_EDGE('',*,*,#5132,.T.);
#7081=ORIENTED_EDGE('',*,*,#5136,.T.);
#7082=ORIENTED_EDGE('',*,*,#5129,.F.);
#7083=ORIENTED_EDGE('',*,*,#5137,.F.);
#7084=ORIENTED_EDGE('',*,*,#5138,.F.);
#7085=ORIENTED_EDGE('',*,*,#5111,.F.);
#7086=ORIENTED_EDGE('',*,*,#5115,.F.);
#7087=ORIENTED_EDGE('',*,*,#5118,.F.);
#7088=ORIENTED_EDGE('',*,*,#5121,.F.);
#7089=ORIENTED_EDGE('',*,*,#5124,.F.);
#7090=ORIENTED_EDGE('',*,*,#5127,.F.);
#7091=ORIENTED_EDGE('',*,*,#5130,.F.);
#7092=ORIENTED_EDGE('',*,*,#5136,.F.);
#7093=ORIENTED_EDGE('',*,*,#5135,.F.);
#7094=ORIENTED_EDGE('',*,*,#5139,.F.);
#7095=ORIENTED_EDGE('',*,*,#5081,.F.);
#7096=ORIENTED_EDGE('',*,*,#5140,.F.);
#7097=ORIENTED_EDGE('',*,*,#5079,.F.);
#7098=ORIENTED_EDGE('',*,*,#5076,.F.);
#7099=ORIENTED_EDGE('',*,*,#5073,.F.);
#7100=ORIENTED_EDGE('',*,*,#5070,.F.);
#7101=ORIENTED_EDGE('',*,*,#5067,.F.);
#7102=ORIENTED_EDGE('',*,*,#5064,.F.);
#7103=ORIENTED_EDGE('',*,*,#5061,.F.);
#7104=ORIENTED_EDGE('',*,*,#5141,.F.);
#7105=ORIENTED_EDGE('',*,*,#5059,.F.);
#7106=ORIENTED_EDGE('',*,*,#5063,.F.);
#7107=ORIENTED_EDGE('',*,*,#5066,.F.);
#7108=ORIENTED_EDGE('',*,*,#5069,.F.);
#7109=ORIENTED_EDGE('',*,*,#5072,.F.);
#7110=ORIENTED_EDGE('',*,*,#5075,.F.);
#7111=ORIENTED_EDGE('',*,*,#5078,.F.);
#7112=ORIENTED_EDGE('',*,*,#5142,.F.);
#7113=ORIENTED_EDGE('',*,*,#5083,.F.);
#7114=ORIENTED_EDGE('',*,*,#5143,.F.);
#7115=ORIENTED_EDGE('',*,*,#5133,.T.);
#7116=ORIENTED_EDGE('',*,*,#5137,.T.);
#7117=ORIENTED_EDGE('',*,*,#5131,.T.);
#7118=ORIENTED_EDGE('',*,*,#5128,.T.);
#7119=ORIENTED_EDGE('',*,*,#5125,.T.);
#7120=ORIENTED_EDGE('',*,*,#5122,.T.);
#7121=ORIENTED_EDGE('',*,*,#5119,.T.);
#7122=ORIENTED_EDGE('',*,*,#5116,.T.);
#7123=ORIENTED_EDGE('',*,*,#5113,.T.);
#7124=ORIENTED_EDGE('',*,*,#5144,.F.);
#7125=ORIENTED_EDGE('',*,*,#5145,.F.);
#7126=ORIENTED_EDGE('',*,*,#5146,.F.);
#7127=ORIENTED_EDGE('',*,*,#5147,.F.);
#7128=ORIENTED_EDGE('',*,*,#5148,.F.);
#7129=ORIENTED_EDGE('',*,*,#5149,.F.);
#7130=ORIENTED_EDGE('',*,*,#5141,.T.);
#7131=ORIENTED_EDGE('',*,*,#5112,.T.);
#7132=ORIENTED_EDGE('',*,*,#5138,.T.);
#7133=ORIENTED_EDGE('',*,*,#5060,.T.);
#7134=ORIENTED_EDGE('',*,*,#5150,.T.);
#7135=ORIENTED_EDGE('',*,*,#5086,.T.);
#7136=ORIENTED_EDGE('',*,*,#5151,.T.);
#7137=ORIENTED_EDGE('',*,*,#5034,.T.);
#7138=ORIENTED_EDGE('',*,*,#5106,.T.);
#7139=ORIENTED_EDGE('',*,*,#5152,.T.);
#7140=ORIENTED_EDGE('',*,*,#5103,.F.);
#7141=ORIENTED_EDGE('',*,*,#5153,.F.);
#7142=ORIENTED_EDGE('',*,*,#5151,.F.);
#7143=ORIENTED_EDGE('',*,*,#5085,.F.);
#7144=ORIENTED_EDGE('',*,*,#5089,.F.);
#7145=ORIENTED_EDGE('',*,*,#5092,.F.);
#7146=ORIENTED_EDGE('',*,*,#5095,.F.);
#7147=ORIENTED_EDGE('',*,*,#5098,.F.);
#7148=ORIENTED_EDGE('',*,*,#5101,.F.);
#7149=ORIENTED_EDGE('',*,*,#5104,.F.);
#7150=ORIENTED_EDGE('',*,*,#5152,.F.);
#7151=ORIENTED_EDGE('',*,*,#5109,.F.);
#7152=ORIENTED_EDGE('',*,*,#5154,.F.);
#7153=ORIENTED_EDGE('',*,*,#5055,.F.);
#7154=ORIENTED_EDGE('',*,*,#5155,.F.);
#7155=ORIENTED_EDGE('',*,*,#5053,.F.);
#7156=ORIENTED_EDGE('',*,*,#5050,.F.);
#7157=ORIENTED_EDGE('',*,*,#5047,.F.);
#7158=ORIENTED_EDGE('',*,*,#5044,.F.);
#7159=ORIENTED_EDGE('',*,*,#5041,.F.);
#7160=ORIENTED_EDGE('',*,*,#5038,.F.);
#7161=ORIENTED_EDGE('',*,*,#5035,.F.);
#7162=ORIENTED_EDGE('',*,*,#5150,.F.);
#7163=ORIENTED_EDGE('',*,*,#5033,.F.);
#7164=ORIENTED_EDGE('',*,*,#5037,.F.);
#7165=ORIENTED_EDGE('',*,*,#5040,.F.);
#7166=ORIENTED_EDGE('',*,*,#5043,.F.);
#7167=ORIENTED_EDGE('',*,*,#5046,.F.);
#7168=ORIENTED_EDGE('',*,*,#5049,.F.);
#7169=ORIENTED_EDGE('',*,*,#5052,.F.);
#7170=ORIENTED_EDGE('',*,*,#5156,.F.);
#7171=ORIENTED_EDGE('',*,*,#5057,.F.);
#7172=ORIENTED_EDGE('',*,*,#5157,.F.);
#7173=ORIENTED_EDGE('',*,*,#5107,.T.);
#7174=ORIENTED_EDGE('',*,*,#5153,.T.);
#7175=ORIENTED_EDGE('',*,*,#5105,.T.);
#7176=ORIENTED_EDGE('',*,*,#5102,.T.);
#7177=ORIENTED_EDGE('',*,*,#5099,.T.);
#7178=ORIENTED_EDGE('',*,*,#5096,.T.);
#7179=ORIENTED_EDGE('',*,*,#5093,.T.);
#7180=ORIENTED_EDGE('',*,*,#5090,.T.);
#7181=ORIENTED_EDGE('',*,*,#5087,.T.);
#7182=ORIENTED_EDGE('',*,*,#5080,.T.);
#7183=ORIENTED_EDGE('',*,*,#5142,.T.);
#7184=ORIENTED_EDGE('',*,*,#5077,.F.);
#7185=ORIENTED_EDGE('',*,*,#5140,.T.);
#7186=ORIENTED_EDGE('',*,*,#5054,.T.);
#7187=ORIENTED_EDGE('',*,*,#5156,.T.);
#7188=ORIENTED_EDGE('',*,*,#5051,.F.);
#7189=ORIENTED_EDGE('',*,*,#5155,.T.);
#7190=ORIENTED_EDGE('',*,*,#5158,.F.);
#7191=ORIENTED_EDGE('',*,*,#5159,.T.);
#7192=ORIENTED_EDGE('',*,*,#5160,.F.);
#7193=ORIENTED_EDGE('',*,*,#5159,.F.);
#7194=ORIENTED_EDGE('',*,*,#5161,.F.);
#7195=ORIENTED_EDGE('',*,*,#5162,.T.);
#7196=ORIENTED_EDGE('',*,*,#5163,.F.);
#7197=ORIENTED_EDGE('',*,*,#5162,.F.);
#7198=ORIENTED_EDGE('',*,*,#5164,.F.);
#7199=ORIENTED_EDGE('',*,*,#5165,.T.);
#7200=ORIENTED_EDGE('',*,*,#5166,.F.);
#7201=ORIENTED_EDGE('',*,*,#5167,.F.);
#7202=ORIENTED_EDGE('',*,*,#5163,.T.);
#7203=ORIENTED_EDGE('',*,*,#5166,.T.);
#7204=ORIENTED_EDGE('',*,*,#5168,.T.);
#7205=ORIENTED_EDGE('',*,*,#5169,.T.);
#7206=ORIENTED_EDGE('',*,*,#5170,.T.);
#7207=ORIENTED_EDGE('',*,*,#5171,.T.);
#7208=ORIENTED_EDGE('',*,*,#5168,.F.);
#7209=ORIENTED_EDGE('',*,*,#5165,.F.);
#7210=ORIENTED_EDGE('',*,*,#5172,.F.);
#7211=ORIENTED_EDGE('',*,*,#5173,.T.);
#7212=ORIENTED_EDGE('',*,*,#5174,.F.);
#7213=ORIENTED_EDGE('',*,*,#5175,.F.);
#7214=ORIENTED_EDGE('',*,*,#5176,.T.);
#7215=ORIENTED_EDGE('',*,*,#5177,.T.);
#7216=ORIENTED_EDGE('',*,*,#5164,.T.);
#7217=ORIENTED_EDGE('',*,*,#5178,.T.);
#7218=ORIENTED_EDGE('',*,*,#5179,.T.);
#7219=ORIENTED_EDGE('',*,*,#5172,.T.);
#7220=ORIENTED_EDGE('',*,*,#5179,.F.);
#7221=ORIENTED_EDGE('',*,*,#5180,.T.);
#7222=ORIENTED_EDGE('',*,*,#5181,.F.);
#7223=ORIENTED_EDGE('',*,*,#5173,.F.);
#7224=ORIENTED_EDGE('',*,*,#5158,.T.);
#7225=ORIENTED_EDGE('',*,*,#5182,.T.);
#7226=ORIENTED_EDGE('',*,*,#5174,.T.);
#7227=ORIENTED_EDGE('',*,*,#5181,.T.);
#7228=ORIENTED_EDGE('',*,*,#5183,.T.);
#7229=ORIENTED_EDGE('',*,*,#5184,.F.);
#7230=ORIENTED_EDGE('',*,*,#5185,.F.);
#7231=ORIENTED_EDGE('',*,*,#5186,.F.);
#7232=ORIENTED_EDGE('',*,*,#5177,.F.);
#7233=ORIENTED_EDGE('',*,*,#5187,.F.);
#7234=ORIENTED_EDGE('',*,*,#5176,.F.);
#7235=ORIENTED_EDGE('',*,*,#5188,.F.);
#7236=ORIENTED_EDGE('',*,*,#5189,.F.);
#7237=ORIENTED_EDGE('',*,*,#5190,.F.);
#7238=ORIENTED_EDGE('',*,*,#5191,.F.);
#7239=ORIENTED_EDGE('',*,*,#5185,.T.);
#7240=ORIENTED_EDGE('',*,*,#5189,.T.);
#7241=ORIENTED_EDGE('',*,*,#5192,.T.);
#7242=ORIENTED_EDGE('',*,*,#5183,.F.);
#7243=ORIENTED_EDGE('',*,*,#5180,.F.);
#7244=ORIENTED_EDGE('',*,*,#5178,.F.);
#7245=ORIENTED_EDGE('',*,*,#5167,.T.);
#7246=ORIENTED_EDGE('',*,*,#5170,.F.);
#7247=ORIENTED_EDGE('',*,*,#5171,.F.);
#7248=ORIENTED_EDGE('',*,*,#5186,.T.);
#7249=ORIENTED_EDGE('',*,*,#5191,.T.);
#7250=ORIENTED_EDGE('',*,*,#5169,.F.);
#7251=ORIENTED_EDGE('',*,*,#5161,.T.);
#7252=ORIENTED_EDGE('',*,*,#5192,.F.);
#7253=ORIENTED_EDGE('',*,*,#5188,.T.);
#7254=ORIENTED_EDGE('',*,*,#5175,.T.);
#7255=ORIENTED_EDGE('',*,*,#5182,.F.);
#7256=ORIENTED_EDGE('',*,*,#5160,.T.);
#7257=ORIENTED_EDGE('',*,*,#5193,.F.);
#7258=ORIENTED_EDGE('',*,*,#5149,.T.);
#7259=ORIENTED_EDGE('',*,*,#5194,.T.);
#7260=ORIENTED_EDGE('',*,*,#5195,.F.);
#7261=ORIENTED_EDGE('',*,*,#5147,.T.);
#7262=ORIENTED_EDGE('',*,*,#5196,.T.);
#7263=ORIENTED_EDGE('',*,*,#5197,.F.);
#7264=ORIENTED_EDGE('',*,*,#5198,.F.);
#7265=ORIENTED_EDGE('',*,*,#5148,.T.);
#7266=ORIENTED_EDGE('',*,*,#5198,.T.);
#7267=ORIENTED_EDGE('',*,*,#5199,.F.);
#7268=ORIENTED_EDGE('',*,*,#5194,.F.);
#7269=ORIENTED_EDGE('',*,*,#5200,.F.);
#7270=ORIENTED_EDGE('',*,*,#5201,.F.);
#7271=ORIENTED_EDGE('',*,*,#5202,.F.);
#7272=ORIENTED_EDGE('',*,*,#5145,.T.);
#7273=ORIENTED_EDGE('',*,*,#5146,.T.);
#7274=ORIENTED_EDGE('',*,*,#5202,.T.);
#7275=ORIENTED_EDGE('',*,*,#5203,.F.);
#7276=ORIENTED_EDGE('',*,*,#5196,.F.);
#7277=ORIENTED_EDGE('',*,*,#5200,.T.);
#7278=ORIENTED_EDGE('',*,*,#5144,.T.);
#7279=ORIENTED_EDGE('',*,*,#5193,.T.);
#7280=ORIENTED_EDGE('',*,*,#5204,.F.);
#7281=ORIENTED_EDGE('',*,*,#5187,.T.);
#7282=ORIENTED_EDGE('',*,*,#5205,.T.);
#7283=ORIENTED_EDGE('',*,*,#5206,.F.);
#7284=ORIENTED_EDGE('',*,*,#5205,.F.);
#7285=ORIENTED_EDGE('',*,*,#5190,.T.);
#7286=ORIENTED_EDGE('',*,*,#5184,.T.);
#7287=ORIENTED_EDGE('',*,*,#5204,.T.);
#7288=ORIENTED_EDGE('',*,*,#5195,.T.);
#7289=ORIENTED_EDGE('',*,*,#5199,.T.);
#7290=ORIENTED_EDGE('',*,*,#5197,.T.);
#7291=ORIENTED_EDGE('',*,*,#5203,.T.);
#7292=ORIENTED_EDGE('',*,*,#5201,.T.);
#7293=ORIENTED_EDGE('',*,*,#5143,.T.);
#7294=ORIENTED_EDGE('',*,*,#5082,.T.);
#7295=ORIENTED_EDGE('',*,*,#5139,.T.);
#7296=ORIENTED_EDGE('',*,*,#5134,.T.);
#7297=ORIENTED_EDGE('',*,*,#5157,.T.);
#7298=ORIENTED_EDGE('',*,*,#5056,.T.);
#7299=ORIENTED_EDGE('',*,*,#5154,.T.);
#7300=ORIENTED_EDGE('',*,*,#5108,.T.);
#7301=ORIENTED_EDGE('',*,*,#5206,.T.);
#8989=CYLINDRICAL_SURFACE('',#10208,0.12645);
#8990=CYLINDRICAL_SURFACE('',#10210,0.12645);
#8991=CYLINDRICAL_SURFACE('',#10211,0.12645);
#8992=CYLINDRICAL_SURFACE('',#10212,0.12645);
#8993=CYLINDRICAL_SURFACE('',#10213,0.12645);
#8994=CYLINDRICAL_SURFACE('',#10214,0.12645);
#8995=CYLINDRICAL_SURFACE('',#10215,0.12645);
#8996=CYLINDRICAL_SURFACE('',#10216,0.12645);
#8997=CYLINDRICAL_SURFACE('',#10218,0.12645);
#8998=CYLINDRICAL_SURFACE('',#10220,0.12645);
#8999=CYLINDRICAL_SURFACE('',#10221,0.12645);
#9000=CYLINDRICAL_SURFACE('',#10222,0.12645);
#9001=CYLINDRICAL_SURFACE('',#10223,0.12645);
#9002=CYLINDRICAL_SURFACE('',#10224,0.12645);
#9003=CYLINDRICAL_SURFACE('',#10225,0.12645);
#9004=CYLINDRICAL_SURFACE('',#10226,0.12645);
#9005=CYLINDRICAL_SURFACE('',#10228,0.1543);
#9006=CYLINDRICAL_SURFACE('',#10230,0.1543);
#9007=CYLINDRICAL_SURFACE('',#10231,0.1543);
#9008=CYLINDRICAL_SURFACE('',#10232,0.1543);
#9009=CYLINDRICAL_SURFACE('',#10233,0.1543);
#9010=CYLINDRICAL_SURFACE('',#10234,0.1543);
#9011=CYLINDRICAL_SURFACE('',#10235,0.1543);
#9012=CYLINDRICAL_SURFACE('',#10236,0.1543);
#9013=CYLINDRICAL_SURFACE('',#10238,0.1543);
#9014=CYLINDRICAL_SURFACE('',#10240,0.1543);
#9015=CYLINDRICAL_SURFACE('',#10241,0.1543);
#9016=CYLINDRICAL_SURFACE('',#10242,0.1543);
#9017=CYLINDRICAL_SURFACE('',#10243,0.1543);
#9018=CYLINDRICAL_SURFACE('',#10244,0.1543);
#9019=CYLINDRICAL_SURFACE('',#10245,0.1543);
#9020=CYLINDRICAL_SURFACE('',#10246,0.1543);
#9021=CYLINDRICAL_SURFACE('',#10248,0.1543);
#9022=CYLINDRICAL_SURFACE('',#10251,0.1543);
#9023=CYLINDRICAL_SURFACE('',#10252,0.12645);
#9024=CYLINDRICAL_SURFACE('',#10253,0.12645);
#9025=CYLINDRICAL_SURFACE('',#10254,0.2);
#9026=CYLINDRICAL_SURFACE('',#10257,0.2);
#9027=CYLINDRICAL_SURFACE('',#10279,1.);
#9028=CYLINDRICAL_SURFACE('',#10281,0.6);
#9406=ADVANCED_FACE('',(#616),#8989,.F.);
#9407=ADVANCED_FACE('',(#617),#8990,.F.);
#9408=ADVANCED_FACE('',(#618),#8991,.F.);
#9409=ADVANCED_FACE('',(#619),#8992,.F.);
#9410=ADVANCED_FACE('',(#620),#8993,.F.);
#9411=ADVANCED_FACE('',(#621),#8994,.F.);
#9412=ADVANCED_FACE('',(#622),#8995,.F.);
#9413=ADVANCED_FACE('',(#623),#8996,.F.);
#9414=ADVANCED_FACE('',(#624),#8997,.F.);
#9415=ADVANCED_FACE('',(#625),#8998,.F.);
#9416=ADVANCED_FACE('',(#626),#8999,.F.);
#9417=ADVANCED_FACE('',(#627),#9000,.F.);
#9418=ADVANCED_FACE('',(#628),#9001,.F.);
#9419=ADVANCED_FACE('',(#629),#9002,.F.);
#9420=ADVANCED_FACE('',(#630),#9003,.F.);
#9421=ADVANCED_FACE('',(#631),#9004,.F.);
#9422=ADVANCED_FACE('',(#632),#9005,.F.);
#9423=ADVANCED_FACE('',(#633),#9006,.F.);
#9424=ADVANCED_FACE('',(#634),#9007,.F.);
#9425=ADVANCED_FACE('',(#635),#9008,.F.);
#9426=ADVANCED_FACE('',(#636),#9009,.F.);
#9427=ADVANCED_FACE('',(#637),#9010,.F.);
#9428=ADVANCED_FACE('',(#638),#9011,.F.);
#9429=ADVANCED_FACE('',(#639),#9012,.F.);
#9430=ADVANCED_FACE('',(#640),#9013,.F.);
#9431=ADVANCED_FACE('',(#641),#9014,.F.);
#9432=ADVANCED_FACE('',(#642),#9015,.F.);
#9433=ADVANCED_FACE('',(#643),#9016,.F.);
#9434=ADVANCED_FACE('',(#644),#9017,.F.);
#9435=ADVANCED_FACE('',(#645),#9018,.F.);
#9436=ADVANCED_FACE('',(#646),#9019,.F.);
#9437=ADVANCED_FACE('',(#647),#9020,.F.);
#9438=ADVANCED_FACE('',(#648),#9021,.F.);
#9439=ADVANCED_FACE('',(#649),#218,.F.);
#9440=ADVANCED_FACE('',(#650),#219,.F.);
#9441=ADVANCED_FACE('',(#651,#267,#268),#342,.F.);
#9442=ADVANCED_FACE('',(#652),#9022,.F.);
#9443=ADVANCED_FACE('',(#653),#220,.F.);
#9444=ADVANCED_FACE('',(#654),#221,.F.);
#9445=ADVANCED_FACE('',(#655),#9023,.F.);
#9446=ADVANCED_FACE('',(#656),#9024,.F.);
#9447=ADVANCED_FACE('',(#657),#9025,.F.);
#9448=ADVANCED_FACE('',(#658),#9026,.F.);
#9449=ADVANCED_FACE('',(#659,#269),#343,.T.);
#9450=ADVANCED_FACE('',(#660),#344,.T.);
#9451=ADVANCED_FACE('',(#661),#345,.T.);
#9452=ADVANCED_FACE('',(#662),#346,.T.);
#9453=ADVANCED_FACE('',(#663,#270),#347,.T.);
#9454=ADVANCED_FACE('',(#664),#348,.T.);
#9455=ADVANCED_FACE('',(#665),#349,.F.);
#9456=ADVANCED_FACE('',(#666),#350,.F.);
#9457=ADVANCED_FACE('',(#667),#351,.T.);
#9458=ADVANCED_FACE('',(#668,#271),#352,.T.);
#9459=ADVANCED_FACE('',(#669,#272),#353,.T.);
#9460=ADVANCED_FACE('',(#670),#354,.T.);
#9461=ADVANCED_FACE('',(#671),#355,.T.);
#9462=ADVANCED_FACE('',(#672),#356,.T.);
#9463=ADVANCED_FACE('',(#673),#357,.T.);
#9464=ADVANCED_FACE('',(#674),#358,.T.);
#9465=ADVANCED_FACE('',(#675),#9027,.T.);
#9466=ADVANCED_FACE('',(#676),#9028,.T.);
#9467=ADVANCED_FACE('',(#677,#273,#274,#275),#359,.T.);
#9770=CLOSED_SHELL('',(#9406,#9407,#9408,#9409,#9410,#9411,#9412,#9413,
#9414,#9415,#9416,#9417,#9418,#9419,#9420,#9421,#9422,#9423,#9424,#9425,
#9426,#9427,#9428,#9429,#9430,#9431,#9432,#9433,#9434,#9435,#9436,#9437,
#9438,#9439,#9440,#9441,#9442,#9443,#9444,#9445,#9446,#9447,#9448,#9449,
#9450,#9451,#9452,#9453,#9454,#9455,#9456,#9457,#9458,#9459,#9460,#9461,
#9462,#9463,#9464,#9465,#9466,#9467));
#10207=AXIS2_PLACEMENT_3D('',#20478,#11345,#11346);
#10208=AXIS2_PLACEMENT_3D('',#20479,#11347,#11348);
#10209=AXIS2_PLACEMENT_3D('',#20489,#11350,#11351);
#10210=AXIS2_PLACEMENT_3D('',#20500,#11352,#11353);
#10211=AXIS2_PLACEMENT_3D('',#20551,#11355,#11356);
#10212=AXIS2_PLACEMENT_3D('',#20602,#11358,#11359);
#10213=AXIS2_PLACEMENT_3D('',#20650,#11361,#11362);
#10214=AXIS2_PLACEMENT_3D('',#20701,#11364,#11365);
#10215=AXIS2_PLACEMENT_3D('',#20752,#11367,#11368);
#10216=AXIS2_PLACEMENT_3D('',#20800,#11370,#11371);
#10217=AXIS2_PLACEMENT_3D('',#20819,#11373,#11374);
#10218=AXIS2_PLACEMENT_3D('',#20839,#11375,#11376);
#10219=AXIS2_PLACEMENT_3D('',#20849,#11378,#11379);
#10220=AXIS2_PLACEMENT_3D('',#20860,#11380,#11381);
#10221=AXIS2_PLACEMENT_3D('',#20911,#11383,#11384);
#10222=AXIS2_PLACEMENT_3D('',#20962,#11386,#11387);
#10223=AXIS2_PLACEMENT_3D('',#21010,#11389,#11390);
#10224=AXIS2_PLACEMENT_3D('',#21061,#11392,#11393);
#10225=AXIS2_PLACEMENT_3D('',#21112,#11395,#11396);
#10226=AXIS2_PLACEMENT_3D('',#21160,#11398,#11399);
#10227=AXIS2_PLACEMENT_3D('',#21179,#11401,#11402);
#10228=AXIS2_PLACEMENT_3D('',#21199,#11403,#11404);
#10229=AXIS2_PLACEMENT_3D('',#21213,#11406,#11407);
#10230=AXIS2_PLACEMENT_3D('',#21223,#11408,#11409);
#10231=AXIS2_PLACEMENT_3D('',#21247,#11411,#11412);
#10232=AXIS2_PLACEMENT_3D('',#21272,#11414,#11415);
#10233=AXIS2_PLACEMENT_3D('',#21297,#11417,#11418);
#10234=AXIS2_PLACEMENT_3D('',#21321,#11420,#11421);
#10235=AXIS2_PLACEMENT_3D('',#21346,#11423,#11424);
#10236=AXIS2_PLACEMENT_3D('',#21371,#11426,#11427);
#10237=AXIS2_PLACEMENT_3D('',#21382,#11429,#11430);
#10238=AXIS2_PLACEMENT_3D('',#21388,#11431,#11432);
#10239=AXIS2_PLACEMENT_3D('',#21402,#11434,#11435);
#10240=AXIS2_PLACEMENT_3D('',#21412,#11436,#11437);
#10241=AXIS2_PLACEMENT_3D('',#21436,#11439,#11440);
#10242=AXIS2_PLACEMENT_3D('',#21461,#11442,#11443);
#10243=AXIS2_PLACEMENT_3D('',#21486,#11445,#11446);
#10244=AXIS2_PLACEMENT_3D('',#21510,#11448,#11449);
#10245=AXIS2_PLACEMENT_3D('',#21535,#11451,#11452);
#10246=AXIS2_PLACEMENT_3D('',#21560,#11454,#11455);
#10247=AXIS2_PLACEMENT_3D('',#21571,#11457,#11458);
#10248=AXIS2_PLACEMENT_3D('',#21577,#11459,#11460);
#10249=AXIS2_PLACEMENT_3D('',#22299,#11461,#11462);
#10250=AXIS2_PLACEMENT_3D('',#22302,#11463,#11464);
#10251=AXIS2_PLACEMENT_3D('',#22413,#11470,#11471);
#10252=AXIS2_PLACEMENT_3D('',#23034,#11472,#11473);
#10253=AXIS2_PLACEMENT_3D('',#23035,#11474,#11475);
#10254=AXIS2_PLACEMENT_3D('',#23036,#11476,#11477);
#10255=AXIS2_PLACEMENT_3D('',#23038,#11478,#11479);
#10256=AXIS2_PLACEMENT_3D('',#23041,#11481,#11482);
#10257=AXIS2_PLACEMENT_3D('',#23042,#11483,#11484);
#10258=AXIS2_PLACEMENT_3D('',#23044,#11485,#11486);
#10259=AXIS2_PLACEMENT_3D('',#23047,#11488,#11489);
#10260=AXIS2_PLACEMENT_3D('',#23048,#11490,#11491);
#10261=AXIS2_PLACEMENT_3D('',#23057,#11496,#11497);
#10262=AXIS2_PLACEMENT_3D('',#23063,#11501,#11502);
#10263=AXIS2_PLACEMENT_3D('',#23077,#11510,#11511);
#10264=AXIS2_PLACEMENT_3D('',#23081,#11514,#11515);
#10265=AXIS2_PLACEMENT_3D('',#23085,#11518,#11519);
#10266=AXIS2_PLACEMENT_3D('',#23089,#11522,#11523);
#10267=AXIS2_PLACEMENT_3D('',#23091,#11524,#11525);
#10268=AXIS2_PLACEMENT_3D('',#23095,#11528,#11529);
#10269=AXIS2_PLACEMENT_3D('',#23097,#11530,#11531);
#10270=AXIS2_PLACEMENT_3D('',#23101,#11534,#11535);
#10271=AXIS2_PLACEMENT_3D('',#23102,#11536,#11537);
#10272=AXIS2_PLACEMENT_3D('',#23105,#11540,#11541);
#10273=AXIS2_PLACEMENT_3D('',#23106,#11542,#11543);
#10274=AXIS2_PLACEMENT_3D('',#23107,#11544,#11545);
#10275=AXIS2_PLACEMENT_3D('',#23113,#11549,#11550);
#10276=AXIS2_PLACEMENT_3D('',#23119,#11554,#11555);
#10277=AXIS2_PLACEMENT_3D('',#23121,#11557,#11558);
#10278=AXIS2_PLACEMENT_3D('',#23127,#11562,#11563);
#10279=AXIS2_PLACEMENT_3D('',#23129,#11565,#11566);
#10280=AXIS2_PLACEMENT_3D('',#23130,#11567,#11568);
#10281=AXIS2_PLACEMENT_3D('',#23131,#11569,#11570);
#10282=AXIS2_PLACEMENT_3D('',#23134,#11572,#11573);
#10283=AXIS2_PLACEMENT_3D('',#23135,#11574,#11575);
#11345=DIRECTION('axis',(0.,0.,1.));
#11346=DIRECTION('refdir',(1.,0.,0.));
#11347=DIRECTION('center_axis',(0.,0.,-1.));
#11348=DIRECTION('ref_axis',(-0.348549200809368,0.937290485716755,0.));
#11349=DIRECTION('',(0.,0.,-1.));
#11350=DIRECTION('center_axis',(0.,0.,-1.));
#11351=DIRECTION('ref_axis',(1.,0.,0.));
#11352=DIRECTION('center_axis',(0.,0.,-1.));
#11353=DIRECTION('ref_axis',(1.,0.,0.));
#11354=DIRECTION('',(0.,0.,-1.));
#11355=DIRECTION('center_axis',(0.,0.,-1.));
#11356=DIRECTION('ref_axis',(1.,0.,0.));
#11357=DIRECTION('',(0.,0.,-1.));
#11358=DIRECTION('center_axis',(0.,0.,-1.));
#11359=DIRECTION('ref_axis',(1.,0.,0.));
#11360=DIRECTION('',(0.,0.,-1.));
#11361=DIRECTION('center_axis',(0.,0.,-1.));
#11362=DIRECTION('ref_axis',(1.,0.,0.));
#11363=DIRECTION('',(0.,0.,-1.));
#11364=DIRECTION('center_axis',(0.,0.,-1.));
#11365=DIRECTION('ref_axis',(1.,0.,0.));
#11366=DIRECTION('',(0.,0.,-1.));
#11367=DIRECTION('center_axis',(0.,0.,-1.));
#11368=DIRECTION('ref_axis',(1.,0.,0.));
#11369=DIRECTION('',(0.,0.,-1.));
#11370=DIRECTION('center_axis',(0.,0.,-1.));
#11371=DIRECTION('ref_axis',(0.93737235570927,-0.348328963412538,0.));
#11372=DIRECTION('',(0.,0.,-1.));
#11373=DIRECTION('center_axis',(0.,0.,-1.));
#11374=DIRECTION('ref_axis',(1.,0.,0.));
#11375=DIRECTION('center_axis',(0.,0.,-1.));
#11376=DIRECTION('ref_axis',(-0.348549399150009,0.937290411960011,0.));
#11377=DIRECTION('',(0.,0.,-1.));
#11378=DIRECTION('center_axis',(0.,0.,-1.));
#11379=DIRECTION('ref_axis',(1.,0.,0.));
#11380=DIRECTION('center_axis',(0.,0.,-1.));
#11381=DIRECTION('ref_axis',(1.,0.,0.));
#11382=DIRECTION('',(0.,0.,-1.));
#11383=DIRECTION('center_axis',(0.,0.,-1.));
#11384=DIRECTION('ref_axis',(1.,0.,0.));
#11385=DIRECTION('',(0.,0.,-1.));
#11386=DIRECTION('center_axis',(0.,0.,-1.));
#11387=DIRECTION('ref_axis',(1.,0.,0.));
#11388=DIRECTION('',(0.,0.,-1.));
#11389=DIRECTION('center_axis',(0.,0.,-1.));
#11390=DIRECTION('ref_axis',(1.,0.,0.));
#11391=DIRECTION('',(0.,0.,-1.));
#11392=DIRECTION('center_axis',(0.,0.,-1.));
#11393=DIRECTION('ref_axis',(1.,0.,0.));
#11394=DIRECTION('',(0.,0.,-1.));
#11395=DIRECTION('center_axis',(0.,0.,-1.));
#11396=DIRECTION('ref_axis',(1.,0.,0.));
#11397=DIRECTION('',(0.,0.,-1.));
#11398=DIRECTION('center_axis',(0.,0.,-1.));
#11399=DIRECTION('ref_axis',(0.937372370252713,-0.348328924275332,0.));
#11400=DIRECTION('',(0.,0.,-1.));
#11401=DIRECTION('center_axis',(0.,0.,-1.));
#11402=DIRECTION('ref_axis',(1.,0.,0.));
#11403=DIRECTION('center_axis',(0.,0.,-1.));
#11404=DIRECTION('ref_axis',(0.793241641674985,0.608906969834288,0.));
#11405=DIRECTION('',(1.22464679914735E-16,-2.74659599554882E-30,-1.));
#11406=DIRECTION('center_axis',(0.,0.,1.));
#11407=DIRECTION('ref_axis',(1.,-2.23051936250031E-14,0.));
#11408=DIRECTION('center_axis',(0.,0.,-1.));
#11409=DIRECTION('ref_axis',(1.,-2.23051936250031E-14,0.));
#11410=DIRECTION('',(1.22464679914735E-16,-2.74659599554882E-30,-1.));
#11411=DIRECTION('center_axis',(0.,0.,-1.));
#11412=DIRECTION('ref_axis',(1.,-2.23051936250031E-14,0.));
#11413=DIRECTION('',(1.22464679914735E-16,-2.74659599554882E-30,-1.));
#11414=DIRECTION('center_axis',(0.,0.,-1.));
#11415=DIRECTION('ref_axis',(1.,-2.23051936250031E-14,0.));
#11416=DIRECTION('',(1.22464679914735E-16,-2.74659599554882E-30,-1.));
#11417=DIRECTION('center_axis',(0.,0.,-1.));
#11418=DIRECTION('ref_axis',(1.,-2.23051936250031E-14,0.));
#11419=DIRECTION('',(1.22464679914735E-16,-2.74659599554882E-30,-1.));
#11420=DIRECTION('center_axis',(0.,0.,-1.));
#11421=DIRECTION('ref_axis',(1.,-2.23051936250031E-14,0.));
#11422=DIRECTION('',(1.22464679914735E-16,-2.74659599554882E-30,-1.));
#11423=DIRECTION('center_axis',(0.,0.,-1.));
#11424=DIRECTION('ref_axis',(1.,-2.23051936250031E-14,0.));
#11425=DIRECTION('',(1.22464679914735E-16,-2.74659599554882E-30,-1.));
#11426=DIRECTION('center_axis',(0.,0.,-1.));
#11427=DIRECTION('ref_axis',(-0.609084174586186,-0.793105584565299,0.));
#11428=DIRECTION('',(1.22464679914735E-16,-2.74659599554882E-30,-1.));
#11429=DIRECTION('center_axis',(0.,0.,-1.));
#11430=DIRECTION('ref_axis',(1.,-2.23051936250031E-14,0.));
#11431=DIRECTION('center_axis',(0.,0.,-1.));
#11432=DIRECTION('ref_axis',(0.793241683023816,0.608906915967904,0.));
#11433=DIRECTION('',(1.22464679914735E-16,-2.65847991820295E-30,-1.));
#11434=DIRECTION('center_axis',(0.,0.,1.));
#11435=DIRECTION('ref_axis',(1.,-2.15856712500031E-14,0.));
#11436=DIRECTION('center_axis',(0.,0.,-1.));
#11437=DIRECTION('ref_axis',(1.,-2.15856712500031E-14,0.));
#11438=DIRECTION('',(1.22464679914735E-16,-2.65847991820295E-30,-1.));
#11439=DIRECTION('center_axis',(0.,0.,-1.));
#11440=DIRECTION('ref_axis',(1.,-2.15856712500031E-14,0.));
#11441=DIRECTION('',(1.22464679914735E-16,-2.65847991820295E-30,-1.));
#11442=DIRECTION('center_axis',(0.,0.,-1.));
#11443=DIRECTION('ref_axis',(1.,-2.15856712500031E-14,0.));
#11444=DIRECTION('',(1.22464679914735E-16,-2.65847991820295E-30,-1.));
#11445=DIRECTION('center_axis',(0.,0.,-1.));
#11446=DIRECTION('ref_axis',(1.,-2.15856712500031E-14,0.));
#11447=DIRECTION('',(1.22464679914735E-16,-2.65847991820295E-30,-1.));
#11448=DIRECTION('center_axis',(0.,0.,-1.));
#11449=DIRECTION('ref_axis',(1.,-2.15856712500031E-14,0.));
#11450=DIRECTION('',(1.22464679914735E-16,-2.65847991820295E-30,-1.));
#11451=DIRECTION('center_axis',(0.,0.,-1.));
#11452=DIRECTION('ref_axis',(1.,-2.15856712500031E-14,0.));
#11453=DIRECTION('',(1.22464679914735E-16,-2.65847991820295E-30,-1.));
#11454=DIRECTION('center_axis',(0.,0.,-1.));
#11455=DIRECTION('ref_axis',(-0.609084235810543,-0.793105537546604,0.));
#11456=DIRECTION('',(1.22464679914735E-16,-2.65847991820295E-30,-1.));
#11457=DIRECTION('center_axis',(0.,0.,-1.));
#11458=DIRECTION('ref_axis',(1.,-2.15856712500031E-14,0.));
#11459=DIRECTION('center_axis',(0.,0.,-1.));
#11460=DIRECTION('ref_axis',(1.,-2.15856712500031E-14,0.));
#11461=DIRECTION('center_axis',(0.,0.,1.));
#11462=DIRECTION('ref_axis',(1.,0.,0.));
#11463=DIRECTION('center_axis',(0.,0.,1.));
#11464=DIRECTION('ref_axis',(1.,0.,0.));
#11465=DIRECTION('',(1.,0.,0.));
#11466=DIRECTION('',(0.,-1.,0.));
#11467=DIRECTION('',(-1.,0.,0.));
#11468=DIRECTION('',(0.,1.,0.));
#11469=DIRECTION('',(1.,0.,0.));
#11470=DIRECTION('center_axis',(0.,0.,-1.));
#11471=DIRECTION('ref_axis',(1.,-2.23051936250031E-14,0.));
#11472=DIRECTION('center_axis',(0.,0.,-1.));
#11473=DIRECTION('ref_axis',(1.,0.,0.));
#11474=DIRECTION('center_axis',(0.,0.,-1.));
#11475=DIRECTION('ref_axis',(1.,0.,0.));
#11476=DIRECTION('center_axis',(-1.,0.,0.));
#11477=DIRECTION('ref_axis',(0.,1.,0.));
#11478=DIRECTION('center_axis',(-1.,0.,0.));
#11479=DIRECTION('ref_axis',(0.,1.,0.));
#11480=DIRECTION('',(-1.,0.,0.));
#11481=DIRECTION('center_axis',(1.,0.,0.));
#11482=DIRECTION('ref_axis',(0.,1.,0.));
#11483=DIRECTION('center_axis',(-1.,0.,0.));
#11484=DIRECTION('ref_axis',(0.,1.,0.));
#11485=DIRECTION('center_axis',(-1.,0.,0.));
#11486=DIRECTION('ref_axis',(0.,1.,0.));
#11487=DIRECTION('',(-1.,0.,0.));
#11488=DIRECTION('center_axis',(1.,0.,0.));
#11489=DIRECTION('ref_axis',(0.,1.,0.));
#11490=DIRECTION('center_axis',(-1.,0.,0.));
#11491=DIRECTION('ref_axis',(0.,-1.,0.));
#11492=DIRECTION('',(0.,1.,0.));
#11493=DIRECTION('',(0.,0.,1.));
#11494=DIRECTION('',(0.,-1.,0.));
#11495=DIRECTION('',(0.,0.,1.));
#11496=DIRECTION('center_axis',(0.,0.,1.));
#11497=DIRECTION('ref_axis',(1.,0.,0.));
#11498=DIRECTION('',(1.,0.,0.));
#11499=DIRECTION('',(0.,1.,0.));
#11500=DIRECTION('',(-1.,0.,0.));
#11501=DIRECTION('center_axis',(0.,-1.,0.));
#11502=DIRECTION('ref_axis',(1.,0.,0.));
#11503=DIRECTION('',(0.,0.,1.));
#11504=DIRECTION('',(1.,0.,0.));
#11505=DIRECTION('',(0.,0.,1.));
#11506=DIRECTION('',(1.,0.,0.));
#11507=DIRECTION('',(0.,0.,1.));
#11508=DIRECTION('',(1.,0.,0.));
#11509=DIRECTION('',(1.,0.,0.));
#11510=DIRECTION('center_axis',(0.,0.,1.));
#11511=DIRECTION('ref_axis',(1.,0.,0.));
#11512=DIRECTION('',(-1.,0.,0.));
#11513=DIRECTION('',(0.,-1.,0.));
#11514=DIRECTION('center_axis',(1.,0.,0.));
#11515=DIRECTION('ref_axis',(0.,1.,0.));
#11516=DIRECTION('',(0.,0.,1.));
#11517=DIRECTION('',(0.,1.,0.));
#11518=DIRECTION('center_axis',(0.,0.,1.));
#11519=DIRECTION('ref_axis',(1.,0.,0.));
#11520=DIRECTION('',(0.,-1.,0.));
#11521=DIRECTION('',(-1.,0.,0.));
#11522=DIRECTION('center_axis',(0.,0.,1.));
#11523=DIRECTION('ref_axis',(1.,0.,0.));
#11524=DIRECTION('center_axis',(0.,0.,-1.));
#11525=DIRECTION('ref_axis',(1.,0.,0.));
#11526=DIRECTION('',(-1.,0.,0.));
#11527=DIRECTION('',(0.,1.,0.));
#11528=DIRECTION('center_axis',(0.,0.,1.));
#11529=DIRECTION('ref_axis',(1.,0.,0.));
#11530=DIRECTION('center_axis',(0.,0.,-1.));
#11531=DIRECTION('ref_axis',(1.,0.,0.));
#11532=DIRECTION('',(0.,-1.,0.));
#11533=DIRECTION('',(-1.,0.,0.));
#11534=DIRECTION('center_axis',(0.,0.,-1.));
#11535=DIRECTION('ref_axis',(1.,0.,0.));
#11536=DIRECTION('center_axis',(0.,1.,0.));
#11537=DIRECTION('ref_axis',(-1.,0.,0.));
#11538=DIRECTION('',(0.,0.,1.));
#11539=DIRECTION('',(0.,0.,1.));
#11540=DIRECTION('center_axis',(1.,0.,0.));
#11541=DIRECTION('ref_axis',(0.,1.,0.));
#11542=DIRECTION('center_axis',(-1.,0.,0.));
#11543=DIRECTION('ref_axis',(0.,-1.,0.));
#11544=DIRECTION('center_axis',(0.,-1.,0.));
#11545=DIRECTION('ref_axis',(1.,0.,0.));
#11546=DIRECTION('',(0.,0.,1.));
#11547=DIRECTION('',(0.,0.,1.));
#11548=DIRECTION('',(1.,0.,0.));
#11549=DIRECTION('center_axis',(0.,1.,0.));
#11550=DIRECTION('ref_axis',(-1.,0.,0.));
#11551=DIRECTION('',(0.,0.,1.));
#11552=DIRECTION('',(-1.,0.,0.));
#11553=DIRECTION('',(0.,0.,1.));
#11554=DIRECTION('center_axis',(1.,0.,0.));
#11555=DIRECTION('ref_axis',(0.,1.,0.));
#11556=DIRECTION('',(0.,1.,0.));
#11557=DIRECTION('center_axis',(0.,-1.,0.));
#11558=DIRECTION('ref_axis',(1.,0.,0.));
#11559=DIRECTION('',(0.,0.,-1.));
#11560=DIRECTION('',(1.,0.,0.));
#11561=DIRECTION('',(0.,0.,1.));
#11562=DIRECTION('center_axis',(-1.,0.,0.));
#11563=DIRECTION('ref_axis',(0.,-1.,0.));
#11564=DIRECTION('',(0.,-1.,0.));
#11565=DIRECTION('center_axis',(0.,0.,1.));
#11566=DIRECTION('ref_axis',(-1.83697019872103E-16,-1.,0.));
#11567=DIRECTION('center_axis',(0.,0.,1.));
#11568=DIRECTION('ref_axis',(1.,0.,0.));
#11569=DIRECTION('center_axis',(0.,0.,1.));
#11570=DIRECTION('ref_axis',(1.,0.,0.));
#11571=DIRECTION('',(0.,0.,-1.));
#11572=DIRECTION('center_axis',(0.,0.,-1.));
#11573=DIRECTION('ref_axis',(1.,0.,0.));
#11574=DIRECTION('center_axis',(0.,0.,1.));
#11575=DIRECTION('ref_axis',(1.,0.,0.));
#20478=CARTESIAN_POINT('',(0.,0.,0.));
#20479=CARTESIAN_POINT('Origin',(0.6,1.,2.15));
#20480=CARTESIAN_POINT('',(0.473748222256554,0.999995809921948,2.01934196736194));
#20481=CARTESIAN_POINT('',(0.473622351265484,0.999839631194249,2.00565803263806));
#20482=CARTESIAN_POINT('',(0.47355,1.,2.15));
#20483=CARTESIAN_POINT('',(0.504188384727762,1.08252112989365,2.));
#20484=CARTESIAN_POINT('Ctrl Pts',(0.473622351265484,0.999839631194249,
2.00565803263806));
#20485=CARTESIAN_POINT('Ctrl Pts',(0.473885391482026,1.02975027328269,2.00377202175871));
#20486=CARTESIAN_POINT('Ctrl Pts',(0.484630619730662,1.05981347843636,2.00188601087935));
#20487=CARTESIAN_POINT('Ctrl Pts',(0.504188384727762,1.08252112989365,2.));
#20488=CARTESIAN_POINT('',(0.695988975197609,1.08263517233072,2.));
#20489=CARTESIAN_POINT('Origin',(0.6,1.,2.));
#20490=CARTESIAN_POINT('Ctrl Pts',(0.69598984030289,1.08263572859344,2.));
#20491=CARTESIAN_POINT('Ctrl Pts',(0.670163701400848,1.11242100165145,2.0024908160387));
#20492=CARTESIAN_POINT('Ctrl Pts',(0.629259702670384,1.12936970915052,2.0049816320774));
#20493=CARTESIAN_POINT('Ctrl Pts',(0.589969605604523,1.12624206673302,2.0074724481161));
#20494=CARTESIAN_POINT('Ctrl Pts',(0.548691445154515,1.12295616684523,2.01008929846199));
#20495=CARTESIAN_POINT('Ctrl Pts',(0.509194644046665,1.09751080441727,2.01270614880789));
#20496=CARTESIAN_POINT('Ctrl Pts',(0.489166147389288,1.06128256435802,2.01532299915378));
#20497=CARTESIAN_POINT('Ctrl Pts',(0.478912868232585,1.04273607706854,2.01666265522317));
#20498=CARTESIAN_POINT('Ctrl Pts',(0.473761783314308,1.02136364588323,2.01800231129256));
#20499=CARTESIAN_POINT('Ctrl Pts',(0.473748222256554,0.999995809921948,
2.01934196736194));
#20500=CARTESIAN_POINT('Origin',(0.6,1.,2.15));
#20501=CARTESIAN_POINT('',(0.473418004372097,0.999922226677399,2.06934196736194));
#20502=CARTESIAN_POINT('',(0.473391518308752,1.00006258785156,2.05565803263806));
#20503=CARTESIAN_POINT('',(0.47355,1.,2.15));
#20504=CARTESIAN_POINT('Ctrl Pts',(0.473391518308752,1.00006258785156,2.05565803263806));
#20505=CARTESIAN_POINT('Ctrl Pts',(0.473368951434719,1.00377931266751,2.05542330751329));
#20506=CARTESIAN_POINT('Ctrl Pts',(0.473518765465857,1.00749417831325,2.05518858238852));
#20507=CARTESIAN_POINT('Ctrl Pts',(0.473846950690071,1.01119320034366,2.05495385726375));
#20508=CARTESIAN_POINT('Ctrl Pts',(0.477505747839885,1.05243201995956,2.05233700691785));
#20509=CARTESIAN_POINT('Ctrl Pts',(0.503334424526069,1.09170162561774,2.04972015657196));
#20510=CARTESIAN_POINT('Ctrl Pts',(0.539751219345993,1.1113984538297,2.04710330622607));
#20511=CARTESIAN_POINT('Ctrl Pts',(0.576168014165918,1.13109528204167,2.04448645588018));
#20512=CARTESIAN_POINT('Ctrl Pts',(0.623172927119585,1.13121933280741,2.04186960553428));
#20513=CARTESIAN_POINT('Ctrl Pts',(0.659688152943108,1.11170438100077,2.03925275518839));
#20514=CARTESIAN_POINT('Ctrl Pts',(0.69620337876663,1.09218942919414,2.0366359048425));
#20515=CARTESIAN_POINT('Ctrl Pts',(0.722228917460009,1.05303547481514,2.0340190544966));
#20516=CARTESIAN_POINT('Ctrl Pts',(0.726095080681017,1.01182045619333,2.03140220415071));
#20517=CARTESIAN_POINT('Ctrl Pts',(0.729961243902025,0.970605437571516,
2.02878535380482));
#20518=CARTESIAN_POINT('Ctrl Pts',(0.711668031650661,0.927329354706896,
2.02616850345893));
#20519=CARTESIAN_POINT('Ctrl Pts',(0.679417475504429,0.901356588462624,
2.02355165311304));
#20520=CARTESIAN_POINT('Ctrl Pts',(0.647166919358198,0.875383822218351,
2.02093480276714));
#20521=CARTESIAN_POINT('Ctrl Pts',(0.600959019317099,0.866714372594425,
2.01831795242125));
#20522=CARTESIAN_POINT('Ctrl Pts',(0.561514908627169,0.879318620323889,
2.01570110207536));
#20523=CARTESIAN_POINT('Ctrl Pts',(0.522070797937238,0.891922868053354,
2.01308425172946));
#20524=CARTESIAN_POINT('Ctrl Pts',(0.489390476598475,0.925800813136209,
2.01046740138357));
#20525=CARTESIAN_POINT('Ctrl Pts',(0.47813574698779,0.965573631142046,2.00785055103768));
#20526=CARTESIAN_POINT('Ctrl Pts',(0.474992502439002,0.976681467377235,
2.00711971157114));
#20527=CARTESIAN_POINT('Ctrl Pts',(0.473520421751905,0.988249094815541,
2.0063888721046));
#20528=CARTESIAN_POINT('Ctrl Pts',(0.473622351265484,0.999839631194249,
2.00565803263806));
#20529=CARTESIAN_POINT('Ctrl Pts',(0.473748222256554,0.999995809921948,
2.01934196736194));
#20530=CARTESIAN_POINT('Ctrl Pts',(0.473735293486444,0.979624254554346,
2.02061916163845));
#20531=CARTESIAN_POINT('Ctrl Pts',(0.478391980488661,0.959256875893503,
2.02189635591496));
#20532=CARTESIAN_POINT('Ctrl Pts',(0.487748897958052,0.941346462457022,
2.02317355019146));
#20533=CARTESIAN_POINT('Ctrl Pts',(0.5069203373911,0.904649718305799,2.02579040053735));
#20534=CARTESIAN_POINT('Ctrl Pts',(0.545823408464101,0.878267347693885,
2.02840725088324));
#20535=CARTESIAN_POINT('Ctrl Pts',(0.587007341569528,0.874020924816605,
2.03102410122914));
#20536=CARTESIAN_POINT('Ctrl Pts',(0.628191274674955,0.869774501939324,
2.03364095157503));
#20537=CARTESIAN_POINT('Ctrl Pts',(0.671656069812808,0.887664026796678,
2.03625780192092));
#20538=CARTESIAN_POINT('Ctrl Pts',(0.697914735578316,0.919671996193035,
2.03887465226682));
#20539=CARTESIAN_POINT('Ctrl Pts',(0.724173401343824,0.951679965589392,
2.04149150261271));
#20540=CARTESIAN_POINT('Ctrl Pts',(0.733225937736988,0.997806379524751,
2.0441083529586));
#20541=CARTESIAN_POINT('Ctrl Pts',(0.72101148240133,1.03736538090912,2.04672520330449));
#20542=CARTESIAN_POINT('Ctrl Pts',(0.708797027065672,1.07692438229349,2.04934205365039));
#20543=CARTESIAN_POINT('Ctrl Pts',(0.675315580001192,1.10991597112687,2.05195890399628));
#20544=CARTESIAN_POINT('Ctrl Pts',(0.635581432895856,1.12154745886576,2.05457575434217));
#20545=CARTESIAN_POINT('Ctrl Pts',(0.59584728579052,1.13317894660465,2.05719260468807));
#20546=CARTESIAN_POINT('Ctrl Pts',(0.549860438644329,1.12345033324905,2.05980945503396));
#20547=CARTESIAN_POINT('Ctrl Pts',(0.518241526751132,1.09672346863534,2.06242630537985));
#20548=CARTESIAN_POINT('Ctrl Pts',(0.490387977892526,1.07317939375162,2.06473152604054));
#20549=CARTESIAN_POINT('Ctrl Pts',(0.473684088301786,1.03644450847376,2.06703674670124));
#20550=CARTESIAN_POINT('Ctrl Pts',(0.473418004372097,0.999922226677399,
2.06934196736194));
#20551=CARTESIAN_POINT('Origin',(0.6,1.,2.15));
#20552=CARTESIAN_POINT('',(0.473569322058917,1.00010891293128,2.11934196736194));
#20553=CARTESIAN_POINT('',(0.473740555540666,1.00002674768131,2.10565803263806));
#20554=CARTESIAN_POINT('',(0.47355,1.,2.15));
#20555=CARTESIAN_POINT('Ctrl Pts',(0.473740555540666,1.00002674768131,2.10565803263806));
#20556=CARTESIAN_POINT('Ctrl Pts',(0.473703568953707,1.01916777914625,2.10445774292198));
#20557=CARTESIAN_POINT('Ctrl Pts',(0.477794964495735,1.03829380542625,2.10325745320589));
#20558=CARTESIAN_POINT('Ctrl Pts',(0.486097635636878,1.0553725521712,2.10205716348981));
#20559=CARTESIAN_POINT('Ctrl Pts',(0.504198971969625,1.09260733284801,2.09944031314392));
#20560=CARTESIAN_POINT('Ctrl Pts',(0.542317321105284,1.12011099531618,2.09682346279803));
#20561=CARTESIAN_POINT('Ctrl Pts',(0.583359964347627,1.12555066422426,2.09420661245214));
#20562=CARTESIAN_POINT('Ctrl Pts',(0.62440260758997,1.13099033313234,2.09158976210624));
#20563=CARTESIAN_POINT('Ctrl Pts',(0.668369544938998,1.11436600848032,2.08897291176035));
#20564=CARTESIAN_POINT('Ctrl Pts',(0.695545474812698,1.08313205071709,2.08635606141446));
#20565=CARTESIAN_POINT('Ctrl Pts',(0.722721404686398,1.05189809295385,2.08373921106856));
#20566=CARTESIAN_POINT('Ctrl Pts',(0.733106327084771,1.00605450207939,2.08112236072267));
#20567=CARTESIAN_POINT('Ctrl Pts',(0.722043527705466,0.966158451314527,
2.07850551037678));
#20568=CARTESIAN_POINT('Ctrl Pts',(0.71098072832616,0.926262400549665,2.07588866003089));
#20569=CARTESIAN_POINT('Ctrl Pts',(0.678470207169174,0.892313889894401,
2.073271809685));
#20570=CARTESIAN_POINT('Ctrl Pts',(0.639090051974211,0.87953512362367,2.0706549593391));
#20571=CARTESIAN_POINT('Ctrl Pts',(0.599709896779248,0.86675635735294,2.06803810899321));
#20572=CARTESIAN_POINT('Ctrl Pts',(0.553460107546307,0.875147335466744,
2.06542125864732));
#20573=CARTESIAN_POINT('Ctrl Pts',(0.52107967173656,0.900946841310449,2.06280440830142));
#20574=CARTESIAN_POINT('Ctrl Pts',(0.491603682429651,0.924432194096951,
2.0604222830803));
#20575=CARTESIAN_POINT('Ctrl Pts',(0.473620539892396,0.962343132242784,
2.05804015785918));
#20576=CARTESIAN_POINT('Ctrl Pts',(0.473391518308752,1.00006258785156,2.05565803263806));
#20577=CARTESIAN_POINT('Ctrl Pts',(0.473418004372097,0.999922226677399,
2.06934196736194));
#20578=CARTESIAN_POINT('Ctrl Pts',(0.473382033997262,0.994984986883897,
2.06965359704714));
#20579=CARTESIAN_POINT('Ctrl Pts',(0.473646461235087,0.990051632376521,
2.06996522673233));
#20580=CARTESIAN_POINT('Ctrl Pts',(0.474224350273596,0.985155275839,2.07027685641753));
#20581=CARTESIAN_POINT('Ctrl Pts',(0.47907706232946,0.944039063528183,2.07289370676342));
#20582=CARTESIAN_POINT('Ctrl Pts',(0.50603346308139,0.905531754778367,2.07551055710931));
#20583=CARTESIAN_POINT('Ctrl Pts',(0.543005874916624,0.886900335416373,
2.0781274074552));
#20584=CARTESIAN_POINT('Ctrl Pts',(0.579978286751859,0.868268916054378,
2.0807442578011));
#20585=CARTESIAN_POINT('Ctrl Pts',(0.626966709670398,0.869513386080205,
2.08336110814699));
#20586=CARTESIAN_POINT('Ctrl Pts',(0.662901030784248,0.890075786233013,
2.08597795849288));
#20587=CARTESIAN_POINT('Ctrl Pts',(0.698835351898097,0.910638186385821,
2.08859480883878));
#20588=CARTESIAN_POINT('Ctrl Pts',(0.723715571207256,0.95051851666561,2.09121165918467));
#20589=CARTESIAN_POINT('Ctrl Pts',(0.726385074899299,0.991833924307951,
2.09382850953056));
#20590=CARTESIAN_POINT('Ctrl Pts',(0.729054578591342,1.03314933195029,2.09644535987645));
#20591=CARTESIAN_POINT('Ctrl Pts',(0.709513366666269,1.07589981695519,2.09906221022235));
#20592=CARTESIAN_POINT('Ctrl Pts',(0.676523964943026,1.10091557332887,2.10167906056824));
#20593=CARTESIAN_POINT('Ctrl Pts',(0.643534563219784,1.12593132970255,2.10429591091413));
#20594=CARTESIAN_POINT('Ctrl Pts',(0.597096971698373,1.13321235744502,2.10691276126002));
#20595=CARTESIAN_POINT('Ctrl Pts',(0.558034351233094,1.1194937471697,2.10952961160592));
#20596=CARTESIAN_POINT('Ctrl Pts',(0.518971730767816,1.10577513689439,2.11214646195181));
#20597=CARTESIAN_POINT('Ctrl Pts',(0.48728408135867,1.0710568886013,2.1147633122977));
#20598=CARTESIAN_POINT('Ctrl Pts',(0.477180525319141,1.0309070826023,2.11738016264359));
#20599=CARTESIAN_POINT('Ctrl Pts',(0.474655708422174,1.02087389149615,2.11803409754971));
#20600=CARTESIAN_POINT('Ctrl Pts',(0.473478752433508,1.01050151615012,2.11868803245583));
#20601=CARTESIAN_POINT('Ctrl Pts',(0.473569322058917,1.00010891293128,2.11934196736194));
#20602=CARTESIAN_POINT('Origin',(0.6,1.,2.15));
#20603=CARTESIAN_POINT('',(0.473701319324768,0.999928563934628,2.16934196736194));
#20604=CARTESIAN_POINT('',(0.473475969746711,0.999901036847401,2.15565803263806));
#20605=CARTESIAN_POINT('',(0.47355,1.,2.15));
#20606=CARTESIAN_POINT('Ctrl Pts',(0.473475969746711,0.999901036847401,
2.15565803263806));
#20607=CARTESIAN_POINT('Ctrl Pts',(0.473771376261924,1.03425627771038,2.15349217833067));
#20608=CARTESIAN_POINT('Ctrl Pts',(0.488302943448428,1.0688317671636,2.15132632402327));
#20609=CARTESIAN_POINT('Ctrl Pts',(0.513274800541643,1.09229629753053,2.14916046971588));
#20610=CARTESIAN_POINT('Ctrl Pts',(0.543446549698046,1.12064684917997,2.14654361936999));
#20611=CARTESIAN_POINT('Ctrl Pts',(0.588859242361366,1.13277740107318,2.1439267690241));
#20612=CARTESIAN_POINT('Ctrl Pts',(0.629149287366476,1.12324847117969,2.1413099186782));
#20613=CARTESIAN_POINT('Ctrl Pts',(0.669439332371586,1.11371954128621,2.13869306833231));
#20614=CARTESIAN_POINT('Ctrl Pts',(0.704606729718486,1.08253112960603,2.13607621798642));
#20615=CARTESIAN_POINT('Ctrl Pts',(0.718882000334445,1.04366848746118,2.13345936764053));
#20616=CARTESIAN_POINT('Ctrl Pts',(0.733157270950405,1.00480584531632,2.13084251729463));
#20617=CARTESIAN_POINT('Ctrl Pts',(0.726540414835423,0.958268972706794,
2.12822566694874));
#20618=CARTESIAN_POINT('Ctrl Pts',(0.701998509069979,0.924925562785253,
2.12560881660285));
#20619=CARTESIAN_POINT('Ctrl Pts',(0.677456603304535,0.891582152863712,
2.12299196625696));
#20620=CARTESIAN_POINT('Ctrl Pts',(0.634989647888627,0.871432205630162,
2.12037511591106));
#20621=CARTESIAN_POINT('Ctrl Pts',(0.59364033014263,0.873511184567866,2.11775826556517));
#20622=CARTESIAN_POINT('Ctrl Pts',(0.552291012396633,0.87559016350557,2.11514141521928));
#20623=CARTESIAN_POINT('Ctrl Pts',(0.512059332320547,0.899898068614528,
2.11252456487339));
#20624=CARTESIAN_POINT('Ctrl Pts',(0.490985654047422,0.935534970611733,
2.10990771452749));
#20625=CARTESIAN_POINT('Ctrl Pts',(0.479577992537903,0.954826036459998,
2.10849115389768));
#20626=CARTESIAN_POINT('Ctrl Pts',(0.473784206454455,0.977436841907783,
2.10707459326787));
#20627=CARTESIAN_POINT('Ctrl Pts',(0.473740555540666,1.00002674768131,2.10565803263806));
#20628=CARTESIAN_POINT('Ctrl Pts',(0.473569322058917,1.00010891293128,2.11934196736194));
#20629=CARTESIAN_POINT('Ctrl Pts',(0.473841184769449,0.968913451231703,
2.12130488280172));
#20630=CARTESIAN_POINT('Ctrl Pts',(0.485533699168036,0.937535732473691,
2.1232677982415));
#20631=CARTESIAN_POINT('Ctrl Pts',(0.506474126044697,0.914602214201428,
2.12523071368127));
#20632=CARTESIAN_POINT('Ctrl Pts',(0.534390745479694,0.884028515504489,
2.12784756402717));
#20633=CARTESIAN_POINT('Ctrl Pts',(0.578743447019601,0.868462481815532,
2.13046441437306));
#20634=CARTESIAN_POINT('Ctrl Pts',(0.619643953027205,0.874884108988649,
2.13308126471895));
#20635=CARTESIAN_POINT('Ctrl Pts',(0.660544459034809,0.881305736161766,
2.13569811506484));
#20636=CARTESIAN_POINT('Ctrl Pts',(0.697992769510109,0.909715024196956,
2.13831496541074));
#20637=CARTESIAN_POINT('Ctrl Pts',(0.715196616413391,0.947372909972802,
2.14093181575663));
#20638=CARTESIAN_POINT('Ctrl Pts',(0.732400463316672,0.985030795748647,
2.14354866610252));
#20639=CARTESIAN_POINT('Ctrl Pts',(0.729359846647935,1.03193727926515,2.14616551644841));
#20640=CARTESIAN_POINT('Ctrl Pts',(0.707438215309595,1.0670589360858,2.14878236679431));
#20641=CARTESIAN_POINT('Ctrl Pts',(0.685516583971256,1.10218059290645,2.1513992171402));
#20642=CARTESIAN_POINT('Ctrl Pts',(0.644713937963314,1.12551742303125,2.15401606748609));
#20643=CARTESIAN_POINT('Ctrl Pts',(0.603326668644815,1.12660491425775,2.15663291783199));
#20644=CARTESIAN_POINT('Ctrl Pts',(0.561939399326316,1.12769240548424,2.15924976817788));
#20645=CARTESIAN_POINT('Ctrl Pts',(0.51996750669726,1.10653055781244,2.16186661852377));
#20646=CARTESIAN_POINT('Ctrl Pts',(0.496231686388225,1.07260859537424,2.16448346886966));
#20647=CARTESIAN_POINT('Ctrl Pts',(0.481542214702607,1.05161518961582,2.16610296836709));
#20648=CARTESIAN_POINT('Ctrl Pts',(0.473837240540682,1.02573460264732,2.16772246786452));
#20649=CARTESIAN_POINT('Ctrl Pts',(0.473701319324768,0.999928563934628,
2.16934196736194));
#20650=CARTESIAN_POINT('Origin',(0.6,1.,2.15));
#20651=CARTESIAN_POINT('',(0.473352235667534,0.999991049382066,2.21934196736194));
#20652=CARTESIAN_POINT('',(0.473504867419963,1.00010483506638,2.20565803263806));
#20653=CARTESIAN_POINT('',(0.47355,1.,2.15));
#20654=CARTESIAN_POINT('Ctrl Pts',(0.473504867419963,1.00010483506638,2.20565803263806));
#20655=CARTESIAN_POINT('Ctrl Pts',(0.473432601452696,1.00827186028206,2.20514346408525));
#20656=CARTESIAN_POINT('Ctrl Pts',(0.474157534286366,1.01642611923938,2.20462889553244));
#20657=CARTESIAN_POINT('Ctrl Pts',(0.475726914006531,1.02441447959464,2.20411432697963));
#20658=CARTESIAN_POINT('Ctrl Pts',(0.48370803108242,1.0650394720171,2.20149747663373));
#20659=CARTESIAN_POINT('Ctrl Pts',(0.513528695332623,1.10137390406913,2.19888062628784));
#20660=CARTESIAN_POINT('Ctrl Pts',(0.551816966436341,1.11712498450026,2.19626377594195));
#20661=CARTESIAN_POINT('Ctrl Pts',(0.59010523754006,1.1328760649314,2.19364692559606));
#20662=CARTESIAN_POINT('Ctrl Pts',(0.636861115497294,1.12804379374164,2.19103007525016));
#20663=CARTESIAN_POINT('Ctrl Pts',(0.671118708852879,1.10479501880275,2.18841322490427));
#20664=CARTESIAN_POINT('Ctrl Pts',(0.705376302208464,1.08154624386386,2.18579637455838));
#20665=CARTESIAN_POINT('Ctrl Pts',(0.7271356109624,1.03988096517584,2.18317952421248));
#20666=CARTESIAN_POINT('Ctrl Pts',(0.726639502419725,0.998482388913484,
2.18056267386659));
#20667=CARTESIAN_POINT('Ctrl Pts',(0.726143393877049,0.95708381265113,2.1779458235207));
#20668=CARTESIAN_POINT('Ctrl Pts',(0.703391868037763,0.915951938814441,
2.17532897317481));
#20669=CARTESIAN_POINT('Ctrl Pts',(0.668586979533722,0.893530788668923,
2.17271212282892));
#20670=CARTESIAN_POINT('Ctrl Pts',(0.63378209102968,0.871109638523405,2.17009527248302));
#20671=CARTESIAN_POINT('Ctrl Pts',(0.586923839860883,0.867399212069058,
2.16747842213713));
#20672=CARTESIAN_POINT('Ctrl Pts',(0.549024022842182,0.88406330841772,2.16486157179124));
#20673=CARTESIAN_POINT('Ctrl Pts',(0.511124205823482,0.900727404766382,
2.16224472144534));
#20674=CARTESIAN_POINT('Ctrl Pts',(0.482182822954877,0.937766023918054,
2.15962787109945));
#20675=CARTESIAN_POINT('Ctrl Pts',(0.475177534345317,0.978570609196729,
2.15701102075356));
#20676=CARTESIAN_POINT('Ctrl Pts',(0.473970221356853,0.985602996945691,
2.15656002471506));
#20677=CARTESIAN_POINT('Ctrl Pts',(0.473414457221305,0.992747241932372,
2.15610902867656));
#20678=CARTESIAN_POINT('Ctrl Pts',(0.473475969746711,0.999901036847401,
2.15565803263806));
#20679=CARTESIAN_POINT('Ctrl Pts',(0.473701319324768,0.999928563934628,
2.16934196736194));
#20680=CARTESIAN_POINT('Ctrl Pts',(0.473617613747686,0.984036200493609,
2.17033931821041));
#20681=CARTESIAN_POINT('Ctrl Pts',(0.476404528994482,0.968172110044866,
2.17133666905888));
#20682=CARTESIAN_POINT('Ctrl Pts',(0.482198594761734,0.953495162034513,
2.17233401990734));
#20683=CARTESIAN_POINT('Ctrl Pts',(0.497401071433289,0.914985768337587,
2.17495087025323));
#20684=CARTESIAN_POINT('Ctrl Pts',(0.533305772765409,0.884649058148337,
2.17756772059913));
#20685=CARTESIAN_POINT('Ctrl Pts',(0.573812603904437,0.876088372947374,
2.18018457094502));
#20686=CARTESIAN_POINT('Ctrl Pts',(0.614319435043466,0.86752768774641,2.18280142129091));
#20687=CARTESIAN_POINT('Ctrl Pts',(0.659428395989404,0.880743027533735,
2.1854182716368));
#20688=CARTESIAN_POINT('Ctrl Pts',(0.688912092443748,0.909808476845009,
2.1880351219827));
#20689=CARTESIAN_POINT('Ctrl Pts',(0.718395788898092,0.938873926156282,
2.19065197232859));
#20690=CARTESIAN_POINT('Ctrl Pts',(0.732254220860843,0.983789484991505,
2.19326882267448));
#20691=CARTESIAN_POINT('Ctrl Pts',(0.724273102711297,1.02441448287903,2.19588567302037));
#20692=CARTESIAN_POINT('Ctrl Pts',(0.716291984561752,1.06503948076655,2.19850252336627));
#20693=CARTESIAN_POINT('Ctrl Pts',(0.686471316299909,1.10137391770637,2.20111937371216));
#20694=CARTESIAN_POINT('Ctrl Pts',(0.648183040045466,1.11712500025644,2.20373622405805));
#20695=CARTESIAN_POINT('Ctrl Pts',(0.609894763791023,1.13287608280652,2.20635307440395));
#20696=CARTESIAN_POINT('Ctrl Pts',(0.563138879543981,1.12804381096685,2.20896992474984));
#20697=CARTESIAN_POINT('Ctrl Pts',(0.528881281579892,1.10479503290036,2.21158677509573));
#20698=CARTESIAN_POINT('Ctrl Pts',(0.49503980248944,1.0818286521973,2.21417183918447));
#20699=CARTESIAN_POINT('Ctrl Pts',(0.473394826320348,1.04089044984514,2.2167569032732));
#20700=CARTESIAN_POINT('Ctrl Pts',(0.473352235667534,0.999991049382066,
2.21934196736194));
#20701=CARTESIAN_POINT('Origin',(0.6,1.,2.15));
#20702=CARTESIAN_POINT('',(0.473682079464411,1.00008273769678,2.26934196736194));
#20703=CARTESIAN_POINT('',(0.473732170341016,0.999958186567598,2.25565803263806));
#20704=CARTESIAN_POINT('',(0.47355,1.,2.15));
#20705=CARTESIAN_POINT('Ctrl Pts',(0.473732170341016,0.999958186567598,
2.25565803263806));
#20706=CARTESIAN_POINT('Ctrl Pts',(0.47380378639699,1.0235579489136,2.25417789949394));
#20707=CARTESIAN_POINT('Ctrl Pts',(0.480162569358453,1.04719354904427,2.25269776634982));
#20708=CARTESIAN_POINT('Ctrl Pts',(0.492561799143745,1.06705892706426,2.25121763320569));
#20709=CARTESIAN_POINT('Ctrl Pts',(0.514483427533268,1.1021805791598,2.2486007828598));
#20710=CARTESIAN_POINT('Ctrl Pts',(0.555286068051798,1.12551740614607,2.24598393251391));
#20711=CARTESIAN_POINT('Ctrl Pts',(0.596673331802579,1.12660489722647,2.24336708216802));
#20712=CARTESIAN_POINT('Ctrl Pts',(0.63806059555336,1.12769238830687,2.24075023182212));
#20713=CARTESIAN_POINT('Ctrl Pts',(0.680032482536391,1.10653054348142,2.23813338147623));
#20714=CARTESIAN_POINT('Ctrl Pts',(0.703768299652422,1.07260858560646,2.23551653113034));
#20715=CARTESIAN_POINT('Ctrl Pts',(0.727504116768454,1.0386866277315,2.23289968078445));
#20716=CARTESIAN_POINT('Ctrl Pts',(0.733003864017485,0.992004556807043,
2.23028283043855));
#20717=CARTESIAN_POINT('Ctrl Pts',(0.717801389391014,0.953495168290641,
2.22766598009266));
#20718=CARTESIAN_POINT('Ctrl Pts',(0.702598914764542,0.914985779774238,
2.22504912974677));
#20719=CARTESIAN_POINT('Ctrl Pts',(0.666694218262566,0.884649073665893,
2.22243227940087));
#20720=CARTESIAN_POINT('Ctrl Pts',(0.626187392572728,0.876088389616529,
2.21981542905498));
#20721=CARTESIAN_POINT('Ctrl Pts',(0.58568056688289,0.867527705567165,2.21719857870909));
#20722=CARTESIAN_POINT('Ctrl Pts',(0.540571612005191,0.880743043576783,
2.2145817283632));
#20723=CARTESIAN_POINT('Ctrl Pts',(0.511087919517129,0.909808488978038,
2.21196487801731));
#20724=CARTESIAN_POINT('Ctrl Pts',(0.487401800053794,0.933158604039368,
2.20986259622422));
#20725=CARTESIAN_POINT('Ctrl Pts',(0.473800111710378,0.966738263555599,
2.20776031443114));
#20726=CARTESIAN_POINT('Ctrl Pts',(0.473504867419963,1.00010483506638,2.20565803263806));
#20727=CARTESIAN_POINT('Ctrl Pts',(0.473352235667534,0.999991049382066,
2.21934196736194));
#20728=CARTESIAN_POINT('Ctrl Pts',(0.473351711967774,0.99948814546325,2.2193737536191));
#20729=CARTESIAN_POINT('Ctrl Pts',(0.473354454431116,0.998985247411069,
2.21940553987625));
#20730=CARTESIAN_POINT('Ctrl Pts',(0.473360480544096,0.998482388709186,
2.21943732613341));
#20731=CARTESIAN_POINT('Ctrl Pts',(0.473856589153524,0.95708380687781,2.2220541764793));
#20732=CARTESIAN_POINT('Ctrl Pts',(0.496608118053516,0.915951927508368,
2.22467102682519));
#20733=CARTESIAN_POINT('Ctrl Pts',(0.531413011239654,0.893530774346426,
2.22728787717109));
#20734=CARTESIAN_POINT('Ctrl Pts',(0.566217904425792,0.871109621184485,
2.22990472751698));
#20735=CARTESIAN_POINT('Ctrl Pts',(0.613076161898077,0.867399194230046,
2.23252157786287));
#20736=CARTESIAN_POINT('Ctrl Pts',(0.650975984015301,0.88406329282086,2.23513842820876));
#20737=CARTESIAN_POINT('Ctrl Pts',(0.688875806132525,0.900727391411673,
2.23775527855466));
#20738=CARTESIAN_POINT('Ctrl Pts',(0.717817192894688,0.93776601554774,2.24037212890055));
#20739=CARTESIAN_POINT('Ctrl Pts',(0.724822482446523,0.978570606314872,
2.24298897924644));
#20740=CARTESIAN_POINT('Ctrl Pts',(0.731827771998358,1.019375197082,2.24560582959233));
#20741=CARTESIAN_POINT('Ctrl Pts',(0.716896964339864,1.0639457544802,2.24822267993823));
#20742=CARTESIAN_POINT('Ctrl Pts',(0.686725211124828,1.09229630994494,2.25083953028412));
#20743=CARTESIAN_POINT('Ctrl Pts',(0.656553457909791,1.12064686540969,2.25345638063001));
#20744=CARTESIAN_POINT('Ctrl Pts',(0.611140759138212,1.13277741894098,2.25607323097591));
#20745=CARTESIAN_POINT('Ctrl Pts',(0.570850708712658,1.12324848776292,2.2586900813218));
#20746=CARTESIAN_POINT('Ctrl Pts',(0.530560658287105,1.11371955658487,2.26130693166769));
#20747=CARTESIAN_POINT('Ctrl Pts',(0.495393256207577,1.08253114069748,2.26392378201358));
#20748=CARTESIAN_POINT('Ctrl Pts',(0.481117983672093,1.04366849332961,2.26654063235948));
#20749=CARTESIAN_POINT('Ctrl Pts',(0.476024096576591,1.02980102162761,2.26747441069363));
#20750=CARTESIAN_POINT('Ctrl Pts',(0.473590398662461,1.01495639211521,2.26840818902779));
#20751=CARTESIAN_POINT('Ctrl Pts',(0.473682079464411,1.00008273769678,2.26934196736194));
#20752=CARTESIAN_POINT('Origin',(0.6,1.,2.15));
#20753=CARTESIAN_POINT('',(0.473597863174539,0.999893075682974,2.31934196736194));
#20754=CARTESIAN_POINT('',(0.473373733146151,0.999953562449677,2.30565803263806));
#20755=CARTESIAN_POINT('',(0.47355,1.,2.15));
#20756=CARTESIAN_POINT('Ctrl Pts',(0.473373733146151,0.999953562449677,
2.30565803263806));
#20757=CARTESIAN_POINT('Ctrl Pts',(0.473559114374899,1.03866557284283,2.30321233490263));
#20758=CARTESIAN_POINT('Ctrl Pts',(0.492644288253083,1.07753593829701,2.3007666371672));
#20759=CARTESIAN_POINT('Ctrl Pts',(0.523476045360312,1.10091555973398,2.29832093943176));
#20760=CARTESIAN_POINT('Ctrl Pts',(0.556465442652399,1.12593131272659,2.29570408908587));
#20761=CARTESIAN_POINT('Ctrl Pts',(0.602903027909946,1.1332123395264,2.29308723873998));
#20762=CARTESIAN_POINT('Ctrl Pts',(0.641965643116553,1.11949373110512,2.29047038839408));
#20763=CARTESIAN_POINT('Ctrl Pts',(0.681028258323161,1.10577512268384,2.28785353804819));
#20764=CARTESIAN_POINT('Ctrl Pts',(0.712715903478828,1.07105687904148,2.2852366877023));
#20765=CARTESIAN_POINT('Ctrl Pts',(0.722819458161278,1.03090707843903,2.28261983735641));
#20766=CARTESIAN_POINT('Ctrl Pts',(0.732923012843728,0.990757277836576,
2.28000298701051));
#20767=CARTESIAN_POINT('Ctrl Pts',(0.72144247705296,0.945175920274039,2.27738613666462));
#20768=CARTESIAN_POINT('Ctrl Pts',(0.693525861372284,0.914602225692484,
2.27476928631873));
#20769=CARTESIAN_POINT('Ctrl Pts',(0.665609245691608,0.88402853111093,2.27215243597284));
#20770=CARTESIAN_POINT('Ctrl Pts',(0.621256550121025,0.868462499510358,
2.26953558562694));
#20771=CARTESIAN_POINT('Ctrl Pts',(0.580356049616192,0.874884125818288,
2.26691873528105));
#20772=CARTESIAN_POINT('Ctrl Pts',(0.539455549111359,0.881305752126219,
2.26430188493516));
#20773=CARTESIAN_POINT('Ctrl Pts',(0.502007243672275,0.909715036342652,
2.26168503458927));
#20774=CARTESIAN_POINT('Ctrl Pts',(0.484803399082991,0.947372917053277,
2.25906818424337));
#20775=CARTESIAN_POINT('Ctrl Pts',(0.477330328981013,0.963730887562828,
2.2579314670416));
#20776=CARTESIAN_POINT('Ctrl Pts',(0.473677170422209,0.981833968538321,
2.25679474983983));
#20777=CARTESIAN_POINT('Ctrl Pts',(0.473732170341016,0.999958186567598,
2.25565803263806));
#20778=CARTESIAN_POINT('Ctrl Pts',(0.473682079464411,1.00008273769678,2.26934196736194));
#20779=CARTESIAN_POINT('Ctrl Pts',(0.473847327881654,0.973273986038867,
2.27102503937368));
#20780=CARTESIAN_POINT('Ctrl Pts',(0.4822169290695,0.946370939387992,2.27270811138542));
#20781=CARTESIAN_POINT('Ctrl Pts',(0.498001477210419,0.924925552697152,
2.27439118339715));
#20782=CARTESIAN_POINT('Ctrl Pts',(0.522543386275672,0.891582138280912,
2.27700803374305));
#20783=CARTESIAN_POINT('Ctrl Pts',(0.565010347397619,0.871432188296782,
2.27962488408894));
#20784=CARTESIAN_POINT('Ctrl Pts',(0.606359670709474,0.873511167531032,
2.28224173443483));
#20785=CARTESIAN_POINT('Ctrl Pts',(0.64770899402133,0.875590146765282,2.28485858478073));
#20786=CARTESIAN_POINT('Ctrl Pts',(0.687940679523094,0.899898055217912,
2.28747543512662));
#20787=CARTESIAN_POINT('Ctrl Pts',(0.709014360624521,0.935534961978321,
2.29009228547251));
#20788=CARTESIAN_POINT('Ctrl Pts',(0.730088041725949,0.971171868738729,
2.2927091358184));
#20789=CARTESIAN_POINT('Ctrl Pts',(0.73200371842704,1.01813777380691,2.2953259861643));
#20790=CARTESIAN_POINT('Ctrl Pts',(0.713902379672349,1.05537255954882,2.29794283651019));
#20791=CARTESIAN_POINT('Ctrl Pts',(0.695801040917658,1.09260734529072,2.30055968685608));
#20792=CARTESIAN_POINT('Ctrl Pts',(0.657682686707185,1.12011101170634,2.30317653720197));
#20793=CARTESIAN_POINT('Ctrl Pts',(0.616640037917562,1.12555068124487,2.30579338754787));
#20794=CARTESIAN_POINT('Ctrl Pts',(0.57559738912794,1.1309903507834,2.30841023789376));
#20795=CARTESIAN_POINT('Ctrl Pts',(0.531630445759169,1.11436602344484,2.31102708823965));
#20796=CARTESIAN_POINT('Ctrl Pts',(0.504454512281174,1.08313206166147,2.31364393858554));
#20797=CARTESIAN_POINT('Ctrl Pts',(0.484729877635794,1.06046205898416,2.31554328151101));
#20798=CARTESIAN_POINT('Ctrl Pts',(0.473850812735054,1.03009564368688,2.31744262443648));
#20799=CARTESIAN_POINT('Ctrl Pts',(0.473597863174539,0.999893075682974,
2.31934196736194));
#20800=CARTESIAN_POINT('Origin',(0.6,1.,2.15));
#20801=CARTESIAN_POINT('',(0.473395817154925,1.00006080538999,2.36934196736194));
#20802=CARTESIAN_POINT('',(0.473630671680838,1.00010094048498,2.35565803263806));
#20803=CARTESIAN_POINT('',(0.47355,1.,2.15));
#20804=CARTESIAN_POINT('',(0.695811615272236,1.08252112989365,2.4));
#20805=CARTESIAN_POINT('Ctrl Pts',(0.473395817154925,1.00006080538999,2.36934196736194));
#20806=CARTESIAN_POINT('Ctrl Pts',(0.473632259557073,0.962556436040281,
2.37171076053695));
#20807=CARTESIAN_POINT('Ctrl Pts',(0.491389033274771,0.924867297705602,
2.37407955371196));
#20808=CARTESIAN_POINT('Ctrl Pts',(0.520582501482215,0.901356555443706,
2.37644834688697));
#20809=CARTESIAN_POINT('Ctrl Pts',(0.552833074551427,0.875383796542954,
2.37906519723286));
#20810=CARTESIAN_POINT('Ctrl Pts',(0.59904103097391,0.866714403531687,2.38168204757875));
#20811=CARTESIAN_POINT('Ctrl Pts',(0.638485120164714,0.879318631335514,
2.38429889792465));
#20812=CARTESIAN_POINT('Ctrl Pts',(0.677929209355517,0.891922859139342,
2.38691574827054));
#20813=CARTESIAN_POINT('Ctrl Pts',(0.710609431314642,0.925800707758264,
2.38953259861643));
#20814=CARTESIAN_POINT('Ctrl Pts',(0.721864159102138,0.965573527992604,
2.39214944896232));
#20815=CARTESIAN_POINT('Ctrl Pts',(0.733118886889633,1.00534634822694,2.39476629930821));
#20816=CARTESIAN_POINT('Ctrl Pts',(0.7229481205055,1.0510141400767,2.39738314965411));
#20817=CARTESIAN_POINT('Ctrl Pts',(0.695811615272236,1.08252112989365,2.4));
#20818=CARTESIAN_POINT('',(0.50401104110406,1.08263520219401,2.4));
#20819=CARTESIAN_POINT('Origin',(0.6,1.,2.4));
#20820=CARTESIAN_POINT('Ctrl Pts',(0.504010178078501,1.08263575731581,2.4));
#20821=CARTESIAN_POINT('Ctrl Pts',(0.529836321312633,1.11242104812743,2.3975091839613));
#20822=CARTESIAN_POINT('Ctrl Pts',(0.57074030629072,1.12936968375571,2.3950183679226));
#20823=CARTESIAN_POINT('Ctrl Pts',(0.610030393987409,1.12624202648756,2.3925275518839));
#20824=CARTESIAN_POINT('Ctrl Pts',(0.651308544594168,1.12295611099769,2.389910701538));
#20825=CARTESIAN_POINT('Ctrl Pts',(0.690805340696773,1.09751079590418,2.38729385119211));
#20826=CARTESIAN_POINT('Ctrl Pts',(0.710833835900798,1.0612825699207,2.38467700084622));
#20827=CARTESIAN_POINT('Ctrl Pts',(0.730862331104824,1.02505434393722,2.38206015050033));
#20828=CARTESIAN_POINT('Ctrl Pts',(0.73142252541027,0.978043207063774,2.37944330015443));
#20829=CARTESIAN_POINT('Ctrl Pts',(0.712251088485857,0.941346462423258,
2.37682644980854));
#20830=CARTESIAN_POINT('Ctrl Pts',(0.693079651561443,0.904649717782742,
2.37420959946265));
#20831=CARTESIAN_POINT('Ctrl Pts',(0.654176583407171,0.878267365375156,
2.37159274911676));
#20832=CARTESIAN_POINT('Ctrl Pts',(0.612992655582392,0.874020946237636,
2.36897589877086));
#20833=CARTESIAN_POINT('Ctrl Pts',(0.571808727757614,0.869774527100117,
2.36635904842497));
#20834=CARTESIAN_POINT('Ctrl Pts',(0.52834394026233,0.887664041232664,2.36374219807908));
#20835=CARTESIAN_POINT('Ctrl Pts',(0.502085278312862,0.919672004499943,
2.36112534773319));
#20836=CARTESIAN_POINT('Ctrl Pts',(0.483798106092066,0.941963130294246,
2.35930290936814));
#20837=CARTESIAN_POINT('Ctrl Pts',(0.473856023642611,0.971101801466951,
2.3574804710031));
#20838=CARTESIAN_POINT('Ctrl Pts',(0.473630671680838,1.00010094048498,2.35565803263806));
#20839=CARTESIAN_POINT('Origin',(-0.6,1.,2.15));
#20840=CARTESIAN_POINT('',(-0.726251764241557,0.999995816438242,2.01934196736194));
#20841=CARTESIAN_POINT('',(-0.726377624507173,0.999839605165841,2.00565803263806));
#20842=CARTESIAN_POINT('',(-0.72645,1.,2.15));
#20843=CARTESIAN_POINT('',(-0.695811615272238,1.08252112989365,2.));
#20844=CARTESIAN_POINT('Ctrl Pts',(-0.726377624507173,0.999839605165841,
2.00565803263806));
#20845=CARTESIAN_POINT('Ctrl Pts',(-0.726114592834244,1.02975025674996,
2.00377202175871));
#20846=CARTESIAN_POINT('Ctrl Pts',(-0.715369380269338,1.05981347843636,
2.00188601087935));
#20847=CARTESIAN_POINT('Ctrl Pts',(-0.695811615272238,1.08252112989365,
2.));
#20848=CARTESIAN_POINT('',(-0.504011038081522,1.08263519664064,2.));
#20849=CARTESIAN_POINT('Origin',(-0.6,1.,2.));
#20850=CARTESIAN_POINT('Ctrl Pts',(-0.504010174669748,1.08263575197435,
2.));
#20851=CARTESIAN_POINT('Ctrl Pts',(-0.529836317100857,1.11242103949754,
2.0024908160387));
#20852=CARTESIAN_POINT('Ctrl Pts',(-0.570740304630068,1.12936968846467,
2.0049816320774));
#20853=CARTESIAN_POINT('Ctrl Pts',(-0.610030394063595,1.12624203395227,
2.0074724481161));
#20854=CARTESIAN_POINT('Ctrl Pts',(-0.651308546495077,1.12295612135759,
2.010089298462));
#20855=CARTESIAN_POINT('Ctrl Pts',(-0.690805343523631,1.09751079747805,
2.01270614880789));
#20856=CARTESIAN_POINT('Ctrl Pts',(-0.710833838996196,1.06128256888394,
2.01532299915378));
#20857=CARTESIAN_POINT('Ctrl Pts',(-0.721087117546352,1.04273608746385,
2.01666265522317));
#20858=CARTESIAN_POINT('Ctrl Pts',(-0.72623820261666,1.02136365505003,2.01800231129255));
#20859=CARTESIAN_POINT('Ctrl Pts',(-0.726251764241557,0.999995816438242,
2.01934196736194));
#20860=CARTESIAN_POINT('Origin',(-0.6,1.,2.15));
#20861=CARTESIAN_POINT('',(-0.7265819818033,0.99992222657182,2.06934196736194));
#20862=CARTESIAN_POINT('',(-0.726608486751216,1.0000625869776,2.05565803263806));
#20863=CARTESIAN_POINT('',(-0.72645,1.,2.15));
#20864=CARTESIAN_POINT('Ctrl Pts',(-0.726608486751216,1.0000625869776,2.05565803263806));
#20865=CARTESIAN_POINT('Ctrl Pts',(-0.726631053637245,1.00377931196893,
2.05542330751329));
#20866=CARTESIAN_POINT('Ctrl Pts',(-0.726481239616099,1.00749417780353,
2.05518858238852));
#20867=CARTESIAN_POINT('Ctrl Pts',(-0.726153054400444,1.01119320003794,
2.05495385726375));
#20868=CARTESIAN_POINT('Ctrl Pts',(-0.722494257346049,1.0524320219281,2.05233700691785));
#20869=CARTESIAN_POINT('Ctrl Pts',(-0.696665580577272,1.09170163174089,
2.04972015657196));
#20870=CARTESIAN_POINT('Ctrl Pts',(-0.660248783717448,1.1113984599152,2.04710330622607));
#20871=CARTESIAN_POINT('Ctrl Pts',(-0.623831986857623,1.13109528808951,
2.04448645588018));
#20872=CARTESIAN_POINT('Ctrl Pts',(-0.576827069906751,1.13121933462535,
2.04186960553428));
#20873=CARTESIAN_POINT('Ctrl Pts',(-0.540311843519016,1.11170438339395,
2.03925275518839));
#20874=CARTESIAN_POINT('Ctrl Pts',(-0.503796617131281,1.09218943216256,
2.0366359048425));
#20875=CARTESIAN_POINT('Ctrl Pts',(-0.477771081306684,1.05303548316395,
2.03401905449661));
#20876=CARTESIAN_POINT('Ctrl Pts',(-0.473904915961309,1.01182046061616,
2.03140220415071));
#20877=CARTESIAN_POINT('Ctrl Pts',(-0.470038750615934,0.970605438068375,
2.02878535380482));
#20878=CARTESIAN_POINT('Ctrl Pts',(-0.48833195574978,0.927329341971419,
2.02616850345893));
#20879=CARTESIAN_POINT('Ctrl Pts',(-0.520582517234745,0.901356578046236,
2.02355165311303));
#20880=CARTESIAN_POINT('Ctrl Pts',(-0.55283307871971,0.875383814121054,
2.02093480276714));
#20881=CARTESIAN_POINT('Ctrl Pts',(-0.599040996555793,0.866714382367644,
2.01831795242125));
#20882=CARTESIAN_POINT('Ctrl Pts',(-0.63848510046728,0.879318623815634,
2.01570110207536));
#20883=CARTESIAN_POINT('Ctrl Pts',(-0.677929204378768,0.891922865263625,
2.01308425172946));
#20884=CARTESIAN_POINT('Ctrl Pts',(-0.710609494365659,0.925800779913016,
2.01046740138357));
#20885=CARTESIAN_POINT('Ctrl Pts',(-0.721864223397342,0.965573598616285,
2.00785055103768));
#20886=CARTESIAN_POINT('Ctrl Pts',(-0.725007467784426,0.976681435046254,
2.00711971157114));
#20887=CARTESIAN_POINT('Ctrl Pts',(-0.726479550710055,0.988249065107503,
2.0063888721046));
#20888=CARTESIAN_POINT('Ctrl Pts',(-0.726377624507173,0.999839605165841,
2.00565803263806));
#20889=CARTESIAN_POINT('Ctrl Pts',(-0.726251764241557,0.999995816438242,
2.01934196736194));
#20890=CARTESIAN_POINT('Ctrl Pts',(-0.726264693552367,0.979624258543708,
2.02061916163845));
#20891=CARTESIAN_POINT('Ctrl Pts',(-0.721608007468156,0.959256876063438,
2.02189635591495));
#20892=CARTESIAN_POINT('Ctrl Pts',(-0.712251090996448,0.941346462433457,
2.02317355019146));
#20893=CARTESIAN_POINT('Ctrl Pts',(-0.693079653607559,0.904649717885772,
2.02579040053735));
#20894=CARTESIAN_POINT('Ctrl Pts',(-0.654176584913204,0.878267362099087,
2.02840725088324));
#20895=CARTESIAN_POINT('Ctrl Pts',(-0.612992656110291,0.874020942267452,
2.03102410122914));
#20896=CARTESIAN_POINT('Ctrl Pts',(-0.571808727307379,0.869774522435818,
2.03364095157503));
#20897=CARTESIAN_POINT('Ctrl Pts',(-0.528343938395909,0.887664038559235,
2.03625780192092));
#20898=CARTESIAN_POINT('Ctrl Pts',(-0.502085275739541,0.919672002962672,
2.03887465226682));
#20899=CARTESIAN_POINT('Ctrl Pts',(-0.475826613083173,0.951679967366109,
2.04149150261271));
#20900=CARTESIAN_POINT('Ctrl Pts',(-0.466774076681907,0.997806380049565,
2.0441083529586));
#20901=CARTESIAN_POINT('Ctrl Pts',(-0.478988530498336,1.03736537794115,
2.04672520330449));
#20902=CARTESIAN_POINT('Ctrl Pts',(-0.491202984314765,1.07692437583273,
2.04934205365039));
#20903=CARTESIAN_POINT('Ctrl Pts',(-0.52468442834889,1.10991595893243,2.05195890399628));
#20904=CARTESIAN_POINT('Ctrl Pts',(-0.564418571222927,1.12154744492272,
2.05457575434217));
#20905=CARTESIAN_POINT('Ctrl Pts',(-0.604152714096964,1.13317893091301,
2.05719260468806));
#20906=CARTESIAN_POINT('Ctrl Pts',(-0.650139555810913,1.12345031979389,
2.05980945503396));
#20907=CARTESIAN_POINT('Ctrl Pts',(-0.681758464159146,1.09672345837341,
2.06242630537985));
#20908=CARTESIAN_POINT('Ctrl Pts',(-0.709612009894941,1.07317938630266,
2.06473152604055));
#20909=CARTESIAN_POINT('Ctrl Pts',(-0.726315897827418,1.03644450458023,
2.06703674670125));
#20910=CARTESIAN_POINT('Ctrl Pts',(-0.7265819818033,0.99992222657182,2.06934196736194));
#20911=CARTESIAN_POINT('Origin',(-0.6,1.,2.15));
#20912=CARTESIAN_POINT('',(-0.726430664085926,1.00010891291408,2.11934196736194));
#20913=CARTESIAN_POINT('',(-0.726259449807842,1.00002674766465,2.10565803263806));
#20914=CARTESIAN_POINT('',(-0.72645,1.,2.15));
#20915=CARTESIAN_POINT('Ctrl Pts',(-0.726259449807842,1.00002674766465,
2.10565803263806));
#20916=CARTESIAN_POINT('Ctrl Pts',(-0.726296436394794,1.01916777993272,
2.10445774292198));
#20917=CARTESIAN_POINT('Ctrl Pts',(-0.722205040678573,1.0382938070189,2.1032574532059));
#20918=CARTESIAN_POINT('Ctrl Pts',(-0.713902369187372,1.05537255449598,
2.10205716348981));
#20919=CARTESIAN_POINT('Ctrl Pts',(-0.695801032091435,1.09260733676896,
2.09944031314392));
#20920=CARTESIAN_POINT('Ctrl Pts',(-0.657682681356665,1.12011100048129,
2.09682346279803));
#20921=CARTESIAN_POINT('Ctrl Pts',(-0.616640036366223,1.12555066958795,
2.09420661245214));
#20922=CARTESIAN_POINT('Ctrl Pts',(-0.57559739137578,1.13099033869461,2.09158976210624));
#20923=CARTESIAN_POINT('Ctrl Pts',(-0.531630452129665,1.1143660131956,2.08897291176035));
#20924=CARTESIAN_POINT('Ctrl Pts',(-0.504454521120231,1.08313205416568,
2.08635606141446));
#20925=CARTESIAN_POINT('Ctrl Pts',(-0.477278590110797,1.05189809513576,
2.08373921106857));
#20926=CARTESIAN_POINT('Ctrl Pts',(-0.466893667338043,1.00605450257494,
2.08112236072267));
#20927=CARTESIAN_POINT('Ctrl Pts',(-0.477956467154043,0.966158450016923,
2.07850551037678));
#20928=CARTESIAN_POINT('Ctrl Pts',(-0.489019266970043,0.926262397458909,
2.07588866003089));
#20929=CARTESIAN_POINT('Ctrl Pts',(-0.521529789374798,0.892313884903708,
2.07327180968499));
#20930=CARTESIAN_POINT('Ctrl Pts',(-0.560909946303062,0.879535118270141,
2.0706549593391));
#20931=CARTESIAN_POINT('Ctrl Pts',(-0.600290103231324,0.866756351636574,
2.06803810899321));
#20932=CARTESIAN_POINT('Ctrl Pts',(-0.646539894683095,0.875147330924641,
2.06542125864732));
#20933=CARTESIAN_POINT('Ctrl Pts',(-0.678920331738974,0.900946837552442,
2.06280440830142));
#20934=CARTESIAN_POINT('Ctrl Pts',(-0.708396322180238,0.924432191052708,
2.0604222830803));
#20935=CARTESIAN_POINT('Ctrl Pts',(-0.726379465045821,0.962343129588992,
2.05804015785918));
#20936=CARTESIAN_POINT('Ctrl Pts',(-0.726608486751216,1.0000625869776,2.05565803263806));
#20937=CARTESIAN_POINT('Ctrl Pts',(-0.7265819818033,0.99992222657182,2.06934196736194));
#20938=CARTESIAN_POINT('Ctrl Pts',(-0.726617952184381,0.99498498729039,
2.06965359704714));
#20939=CARTESIAN_POINT('Ctrl Pts',(-0.726353524983949,0.990051633299336,
2.06996522673233));
#20940=CARTESIAN_POINT('Ctrl Pts',(-0.725775636014574,0.985155277281126,
2.07027685641753));
#20941=CARTESIAN_POINT('Ctrl Pts',(-0.720922924539255,0.944039069331128,
2.07289370676342));
#20942=CARTESIAN_POINT('Ctrl Pts',(-0.693966526606102,0.905531765152948,
2.07551055710931));
#20943=CARTESIAN_POINT('Ctrl Pts',(-0.656994118794319,0.886900347913169,
2.0781274074552));
#20944=CARTESIAN_POINT('Ctrl Pts',(-0.620021710982536,0.868268930673389,
2.0807442578011));
#20945=CARTESIAN_POINT('Ctrl Pts',(-0.573033293292122,0.86951340037201,
2.08336110814699));
#20946=CARTESIAN_POINT('Ctrl Pts',(-0.537098976133817,0.890075798227289,
2.08597795849288));
#20947=CARTESIAN_POINT('Ctrl Pts',(-0.501164658975514,0.910638196082568,
2.08859480883878));
#20948=CARTESIAN_POINT('Ctrl Pts',(-0.476284442349319,0.950518522094504,
2.09121165918467));
#20949=CARTESIAN_POINT('Ctrl Pts',(-0.473614938940181,0.991833925232179,
2.09382850953056));
#20950=CARTESIAN_POINT('Ctrl Pts',(-0.470945435531044,1.03314932836985,
2.09644535987645));
#20951=CARTESIAN_POINT('Ctrl Pts',(-0.490486645338963,1.07589980863327,
2.09906221022235));
#20952=CARTESIAN_POINT('Ctrl Pts',(-0.523476043451828,1.10091556225217,
2.10167906056824));
#20953=CARTESIAN_POINT('Ctrl Pts',(-0.556465441564692,1.12593131587107,
2.10429591091413));
#20954=CARTESIAN_POINT('Ctrl Pts',(-0.6029030279825,1.13321234284545,2.10691276126002));
#20955=CARTESIAN_POINT('Ctrl Pts',(-0.64196564416317,1.11949373408075,2.10952961160592));
#20956=CARTESIAN_POINT('Ctrl Pts',(-0.68102826034384,1.10577512531604,2.11214646195181));
#20957=CARTESIAN_POINT('Ctrl Pts',(-0.712715906287371,1.07105688081224,
2.1147633122977));
#20958=CARTESIAN_POINT('Ctrl Pts',(-0.722819461221189,1.03090707921019,
2.1173801626436));
#20959=CARTESIAN_POINT('Ctrl Pts',(-0.725344277841846,1.02087388920281,
2.11803409754971));
#20960=CARTESIAN_POINT('Ctrl Pts',(-0.72652123370157,1.01050151499351,2.11868803245583));
#20961=CARTESIAN_POINT('Ctrl Pts',(-0.726430664085926,1.00010891291408,
2.11934196736194));
#20962=CARTESIAN_POINT('Origin',(-0.6,1.,2.15));
#20963=CARTESIAN_POINT('',(-0.726298666832045,0.999928563942421,2.16934196736194));
#20964=CARTESIAN_POINT('',(-0.72652403561687,0.999901036843312,2.15565803263806));
#20965=CARTESIAN_POINT('',(-0.72645,1.,2.15));
#20966=CARTESIAN_POINT('Ctrl Pts',(-0.72652403561687,0.999901036843312,
2.15565803263806));
#20967=CARTESIAN_POINT('Ctrl Pts',(-0.726228629089082,1.03425627916229,
2.15349217833067));
#20968=CARTESIAN_POINT('Ctrl Pts',(-0.711697061286474,1.06883177008057,
2.15132632402327));
#20969=CARTESIAN_POINT('Ctrl Pts',(-0.686725203134716,1.09229630144258,
2.14916046971588));
#20970=CARTESIAN_POINT('Ctrl Pts',(-0.65655345269935,1.12064685429431,2.14654361936999));
#20971=CARTESIAN_POINT('Ctrl Pts',(-0.611140758111187,1.13277740670372,
2.1439267690241));
#20972=CARTESIAN_POINT('Ctrl Pts',(-0.570850711397976,1.12324847640543,
2.1413099186782));
#20973=CARTESIAN_POINT('Ctrl Pts',(-0.530560664684765,1.11371954610715,
2.13869306833231));
#20974=CARTESIAN_POINT('Ctrl Pts',(-0.495393265846508,1.08253113310118,
2.13607621798642));
#20975=CARTESIAN_POINT('Ctrl Pts',(-0.481117994625666,1.04366848931044,
2.13345936764053));
#20976=CARTESIAN_POINT('Ctrl Pts',(-0.466842723404823,1.00480584551971,
2.13084251729463));
#20977=CARTESIAN_POINT('Ctrl Pts',(-0.473459579801396,0.958268970944215,
2.12822566694874));
#20978=CARTESIAN_POINT('Ctrl Pts',(-0.498001486606679,0.924925559606287,
2.12560881660285));
#20979=CARTESIAN_POINT('Ctrl Pts',(-0.522543393411961,0.89158214826836,
2.12299196625695));
#20980=CARTESIAN_POINT('Ctrl Pts',(-0.565010350625955,0.871432200167998,
2.12037511591106));
#20981=CARTESIAN_POINT('Ctrl Pts',(-0.606359670125879,0.873511179199166,
2.11775826556517));
#20982=CARTESIAN_POINT('Ctrl Pts',(-0.647708989625804,0.875590158230334,
2.11514141521928));
#20983=CARTESIAN_POINT('Ctrl Pts',(-0.687940671411661,0.899898064393031,
2.11252456487338));
#20984=CARTESIAN_POINT('Ctrl Pts',(-0.709014350576037,0.935534967891196,
2.10990771452749));
#20985=CARTESIAN_POINT('Ctrl Pts',(-0.72042201256801,0.954826034551965,
2.10849115389768));
#20986=CARTESIAN_POINT('Ctrl Pts',(-0.726215798894061,0.977436840943303,
2.10707459326787));
#20987=CARTESIAN_POINT('Ctrl Pts',(-0.726259449807842,1.00002674766465,
2.10565803263806));
#20988=CARTESIAN_POINT('Ctrl Pts',(-0.726430664085926,1.00010891291408,
2.11934196736194));
#20989=CARTESIAN_POINT('Ctrl Pts',(-0.726158801404701,0.968913454634673,
2.12130488280172));
#20990=CARTESIAN_POINT('Ctrl Pts',(-0.714466288285182,0.937535739321086,
2.1232677982415));
#20991=CARTESIAN_POINT('Ctrl Pts',(-0.693525863703029,0.914602223563998,
2.12523071368127));
#20992=CARTESIAN_POINT('Ctrl Pts',(-0.665609247326942,0.884028528220152,
2.12784756402716));
#20993=CARTESIAN_POINT('Ctrl Pts',(-0.621256550650662,0.868462496232756,
2.13046441437306));
#20994=CARTESIAN_POINT('Ctrl Pts',(-0.580356049126553,0.874884122700947,
2.13308126471895));
#20995=CARTESIAN_POINT('Ctrl Pts',(-0.539455547602445,0.881305749169137,
2.13569811506484));
#20996=CARTESIAN_POINT('Ctrl Pts',(-0.502007241230509,0.909715034092914,
2.13831496541074));
#20997=CARTESIAN_POINT('Ctrl Pts',(-0.484803396212605,0.947372915741768,
2.14093181575663));
#20998=CARTESIAN_POINT('Ctrl Pts',(-0.467599551194702,0.985030797390621,
2.14354866610252));
#20999=CARTESIAN_POINT('Ctrl Pts',(-0.470640167530832,1.03193727576455,
2.14616551644841));
#21000=CARTESIAN_POINT('Ctrl Pts',(-0.492561796466562,1.06705892873532,
2.14878236679431));
#21001=CARTESIAN_POINT('Ctrl Pts',(-0.514483425402293,1.10218058170609,
2.1513992171402));
#21002=CARTESIAN_POINT('Ctrl Pts',(-0.555286066937625,1.1255174092737,2.15401606748609));
#21003=CARTESIAN_POINT('Ctrl Pts',(-0.596673331719711,1.12660490038116,
2.15663291783198));
#21004=CARTESIAN_POINT('Ctrl Pts',(-0.638060596501796,1.12769239148863,
2.15924976817788));
#21005=CARTESIAN_POINT('Ctrl Pts',(-0.680032484530636,1.10653054613594,
2.16186661852377));
#21006=CARTESIAN_POINT('Ctrl Pts',(-0.703768302238105,1.07260858741574,
2.16448346886966));
#21007=CARTESIAN_POINT('Ctrl Pts',(-0.718457772313683,1.05161518395829,
2.16610296836709));
#21008=CARTESIAN_POINT('Ctrl Pts',(-0.726162745631061,1.02573459982654,
2.16772246786452));
#21009=CARTESIAN_POINT('Ctrl Pts',(-0.726298666832045,0.999928563942421,
2.16934196736194));
#21010=CARTESIAN_POINT('Origin',(-0.6,1.,2.15));
#21011=CARTESIAN_POINT('',(-0.726647750450984,0.999991049383163,2.21934196736194));
#21012=CARTESIAN_POINT('',(-0.726495137942383,1.00010483507083,2.20565803263806));
#21013=CARTESIAN_POINT('',(-0.72645,1.,2.15));
#21014=CARTESIAN_POINT('Ctrl Pts',(-0.726495137942383,1.00010483507083,
2.20565803263806));
#21015=CARTESIAN_POINT('Ctrl Pts',(-0.726567403912713,1.00827186063272,
2.20514346408525));
#21016=CARTESIAN_POINT('Ctrl Pts',(-0.725842471048314,1.01642611993573,
2.20462889553244));
#21017=CARTESIAN_POINT('Ctrl Pts',(-0.72427309126162,1.02441448062962,2.20411432697963));
#21018=CARTESIAN_POINT('Ctrl Pts',(-0.716291973847398,1.06503947477424,
2.20149747663373));
#21019=CARTESIAN_POINT('Ctrl Pts',(-0.686471308333041,1.10137390836652,
2.19888062628784));
#21020=CARTESIAN_POINT('Ctrl Pts',(-0.648183035606218,1.11712498946538,
2.19626377594195));
#21021=CARTESIAN_POINT('Ctrl Pts',(-0.609894762879395,1.13287607056424,
2.19364692559606));
#21022=CARTESIAN_POINT('Ctrl Pts',(-0.563138882940105,1.12804379916968,
2.19103007525017));
#21023=CARTESIAN_POINT('Ctrl Pts',(-0.52888128813228,1.10479502324521,2.18841322490427));
#21024=CARTESIAN_POINT('Ctrl Pts',(-0.494623693324455,1.08154624732075,
2.18579637455838));
#21025=CARTESIAN_POINT('Ctrl Pts',(-0.472864383648094,1.03988096686638,
2.18317952421249));
#21026=CARTESIAN_POINT('Ctrl Pts',(-0.473360492211805,0.998482388849106,
2.18056267386659));
#21027=CARTESIAN_POINT('Ctrl Pts',(-0.473856600775515,0.957083810831832,
2.1779458235207));
#21028=CARTESIAN_POINT('Ctrl Pts',(-0.496608127579297,0.915951935251654,
2.17532897317481));
#21029=CARTESIAN_POINT('Ctrl Pts',(-0.531413017558768,0.893530784155595,
2.17271212282892));
#21030=CARTESIAN_POINT('Ctrl Pts',(-0.56621790753824,0.871109633059536,
2.17009527248302));
#21031=CARTESIAN_POINT('Ctrl Pts',(-0.613076160693402,0.867399206447596,
2.16747842213713));
#21032=CARTESIAN_POINT('Ctrl Pts',(-0.650975979318758,0.884063303502809,
2.16486157179124));
#21033=CARTESIAN_POINT('Ctrl Pts',(-0.688875797944115,0.900727400558021,
2.16224472144534));
#21034=CARTESIAN_POINT('Ctrl Pts',(-0.717817182039666,0.937766021280388,
2.15962787109945));
#21035=CARTESIAN_POINT('Ctrl Pts',(-0.724822470946157,0.978570608288594,
2.15701102075356));
#21036=CARTESIAN_POINT('Ctrl Pts',(-0.726029783985795,0.985602996335628,
2.15656002471506));
#21037=CARTESIAN_POINT('Ctrl Pts',(-0.726585548144894,0.9927472416251,2.15610902867656));
#21038=CARTESIAN_POINT('Ctrl Pts',(-0.72652403561687,0.999901036843312,
2.15565803263806));
#21039=CARTESIAN_POINT('Ctrl Pts',(-0.726298666832045,0.999928563942421,
2.16934196736194));
#21040=CARTESIAN_POINT('Ctrl Pts',(-0.726382372399933,0.984036202243351,
2.17033931821041));
#21041=CARTESIAN_POINT('Ctrl Pts',(-0.723595457458582,0.968172113533461,
2.17133666905888));
#21042=CARTESIAN_POINT('Ctrl Pts',(-0.71780139232639,0.95349516713182,2.17233401990734));
#21043=CARTESIAN_POINT('Ctrl Pts',(-0.702598917321108,0.914985777655832,
2.17495087025323));
#21044=CARTESIAN_POINT('Ctrl Pts',(-0.666694219924447,0.884649070791584,
2.17756772059913));
#21045=CARTESIAN_POINT('Ctrl Pts',(-0.626187393225259,0.876088386528911,
2.18018457094502));
#21046=CARTESIAN_POINT('Ctrl Pts',(-0.58568056652607,0.867527702266238,
2.18280142129091));
#21047=CARTESIAN_POINT('Ctrl Pts',(-0.540571610524354,0.880743040605142,
2.1854182716368));
#21048=CARTESIAN_POINT('Ctrl Pts',(-0.511087917301621,0.909808486730647,
2.1880351219827));
#21049=CARTESIAN_POINT('Ctrl Pts',(-0.481604224078888,0.938873932856152,
2.19065197232859));
#21050=CARTESIAN_POINT('Ctrl Pts',(-0.467745793635136,0.983789486768259,
2.19326882267448));
#21051=CARTESIAN_POINT('Ctrl Pts',(-0.475726910909899,1.02441448020301,
2.19588567302037));
#21052=CARTESIAN_POINT('Ctrl Pts',(-0.483708028184661,1.06503947363776,
2.19850252336627));
#21053=CARTESIAN_POINT('Ctrl Pts',(-0.513528693177939,1.10137390659515,
2.20111937371216));
#21054=CARTESIAN_POINT('Ctrl Pts',(-0.551816965235723,1.11712498741877,
2.20373622405805));
#21055=CARTESIAN_POINT('Ctrl Pts',(-0.590105237293507,1.1328760682424,2.20635307440395));
#21056=CARTESIAN_POINT('Ctrl Pts',(-0.636861116415798,1.12804379693225,
2.20896992474984));
#21057=CARTESIAN_POINT('Ctrl Pts',(-0.671118710625013,1.10479502141404,
2.21158677509573));
#21058=CARTESIAN_POINT('Ctrl Pts',(-0.704960186006201,1.0818286432283,2.21417183918447));
#21059=CARTESIAN_POINT('Ctrl Pts',(-0.726605159802828,1.04089044536347,
2.21675690327321));
#21060=CARTESIAN_POINT('Ctrl Pts',(-0.726647750450984,0.999991049383163,
2.21934196736194));
#21061=CARTESIAN_POINT('Origin',(-0.6,1.,2.15));
#21062=CARTESIAN_POINT('',(-0.726317906690824,1.0000827376849,2.26934196736194));
#21063=CARTESIAN_POINT('',(-0.726267835011577,0.999958186565595,2.25565803263806));
#21064=CARTESIAN_POINT('',(-0.72645,1.,2.15));
#21065=CARTESIAN_POINT('Ctrl Pts',(-0.726267835011577,0.999958186565595,
2.25565803263806));
#21066=CARTESIAN_POINT('Ctrl Pts',(-0.726196218952626,1.02355794991214,
2.25417789949394));
#21067=CARTESIAN_POINT('Ctrl Pts',(-0.719837435721701,1.04719355104496,
2.25269776634982));
#21068=CARTESIAN_POINT('Ctrl Pts',(-0.707438205410818,1.06705892990714,
2.25121763320569));
#21069=CARTESIAN_POINT('Ctrl Pts',(-0.685516576092059,1.10218058349167,
2.2486007828598));
#21070=CARTESIAN_POINT('Ctrl Pts',(-0.644713933843695,1.12551741146695,
2.24598393251391));
#21071=CARTESIAN_POINT('Ctrl Pts',(-0.603326668338405,1.12660490259339,
2.24336708216802));
#21072=CARTESIAN_POINT('Ctrl Pts',(-0.561939402833115,1.12769239371984,
2.24075023182213));
#21073=CARTESIAN_POINT('Ctrl Pts',(-0.519967514070899,1.10653054799744,
2.23813338147623));
#21074=CARTESIAN_POINT('Ctrl Pts',(-0.496231695948683,1.0726085886845,2.23551653113034));
#21075=CARTESIAN_POINT('Ctrl Pts',(-0.472495877826467,1.03868662937157,
2.23289968078445));
#21076=CARTESIAN_POINT('Ctrl Pts',(-0.466996130344251,0.992004556468098,
2.23028283043855));
#21077=CARTESIAN_POINT('Ctrl Pts',(-0.482198605615172,0.9534951663192,2.22766598009266));
#21078=CARTESIAN_POINT('Ctrl Pts',(-0.497401080886093,0.914985776170301,
2.22504912974677));
#21079=CARTESIAN_POINT('Ctrl Pts',(-0.533305778910153,0.884649068775973,
2.22243227940087));
#21080=CARTESIAN_POINT('Ctrl Pts',(-0.573812606317149,0.876088384363716,
2.21981542905498));
#21081=CARTESIAN_POINT('Ctrl Pts',(-0.614319433724146,0.867527699951458,
2.21719857870909));
#21082=CARTESIAN_POINT('Ctrl Pts',(-0.659428390514079,0.88074303852127,
2.2145817283632));
#21083=CARTESIAN_POINT('Ctrl Pts',(-0.688912084252003,0.909808485154657,
2.21196487801731));
#21084=CARTESIAN_POINT('Ctrl Pts',(-0.712598204719431,0.933158601205837,
2.20986259622422));
#21085=CARTESIAN_POINT('Ctrl Pts',(-0.72619989363945,0.96673826214558,2.20776031443114));
#21086=CARTESIAN_POINT('Ctrl Pts',(-0.726495137942383,1.00010483507083,
2.20565803263806));
#21087=CARTESIAN_POINT('Ctrl Pts',(-0.726647750450984,0.999991049383163,
2.21934196736194));
#21088=CARTESIAN_POINT('Ctrl Pts',(-0.726648274150687,0.999488145519468,
2.2193737536191));
#21089=CARTESIAN_POINT('Ctrl Pts',(-0.726645531687645,0.998985247522407,
2.21940553987625));
#21090=CARTESIAN_POINT('Ctrl Pts',(-0.726639505575326,0.99848238887564,
2.21943732613341));
#21091=CARTESIAN_POINT('Ctrl Pts',(-0.726143397020285,0.957083811581739,
2.2220541764793));
#21092=CARTESIAN_POINT('Ctrl Pts',(-0.703391870614066,0.915951936720223,
2.22467102682519));
#21093=CARTESIAN_POINT('Ctrl Pts',(-0.668586981242762,0.893530786015975,
2.22728787717108));
#21094=CARTESIAN_POINT('Ctrl Pts',(-0.633782091871458,0.871109635311727,
2.22990472751698));
#21095=CARTESIAN_POINT('Ctrl Pts',(-0.586923839535069,0.867399208764748,
2.23252157786287));
#21096=CARTESIAN_POINT('Ctrl Pts',(-0.549024021571972,0.884063305528724,
2.23513842820877));
#21097=CARTESIAN_POINT('Ctrl Pts',(-0.511124203608875,0.9007274022927,2.23775527855466));
#21098=CARTESIAN_POINT('Ctrl Pts',(-0.48218282001907,0.93776602236763,2.24037212890055));
#21099=CARTESIAN_POINT('Ctrl Pts',(-0.475177531234974,0.978570608662929,
2.24298897924644));
#21100=CARTESIAN_POINT('Ctrl Pts',(-0.468172242450878,1.01937519495823,
2.24560582959233));
#21101=CARTESIAN_POINT('Ctrl Pts',(-0.483103048472492,1.06394574747389,
2.24822267993823));
#21102=CARTESIAN_POINT('Ctrl Pts',(-0.513274798380673,1.09229629983004,
2.25083953028412));
#21103=CARTESIAN_POINT('Ctrl Pts',(-0.543446548288854,1.12064685218619,
2.25345638063001));
#21104=CARTESIAN_POINT('Ctrl Pts',(-0.588859242083601,1.13277740438282,
2.25607323097591));
#21105=CARTESIAN_POINT('Ctrl Pts',(-0.629149288092737,1.1232484742514,2.2586900813218));
#21106=CARTESIAN_POINT('Ctrl Pts',(-0.669439334101873,1.11371954411997,
2.26130693166769));
#21107=CARTESIAN_POINT('Ctrl Pts',(-0.704606732325397,1.08253113166048,
2.26392378201358));
#21108=CARTESIAN_POINT('Ctrl Pts',(-0.718882003296907,1.04366848854818,
2.26654063235948));
#21109=CARTESIAN_POINT('Ctrl Pts',(-0.723975889834331,1.0298010183647,2.26747441069363));
#21110=CARTESIAN_POINT('Ctrl Pts',(-0.726409587482227,1.01495639047621,
2.26840818902779));
#21111=CARTESIAN_POINT('Ctrl Pts',(-0.726317906690824,1.0000827376849,2.26934196736194));
#21112=CARTESIAN_POINT('Origin',(-0.6,1.,2.15));
#21113=CARTESIAN_POINT('',(-0.72640212307541,0.999893075304641,2.31934196736194));
#21114=CARTESIAN_POINT('',(-0.726626272216059,0.999953562434948,2.30565803263806));
#21115=CARTESIAN_POINT('',(-0.72645,1.,2.15));
#21116=CARTESIAN_POINT('Ctrl Pts',(-0.726626272216059,0.999953562434948,
2.30565803263806));
#21117=CARTESIAN_POINT('Ctrl Pts',(-0.726440890977488,1.03866557446413,
2.30321233490263));
#21118=CARTESIAN_POINT('Ctrl Pts',(-0.707355716298753,1.0775359415853,2.3007666371672));
#21119=CARTESIAN_POINT('Ctrl Pts',(-0.676523957886503,1.10091556401805,
2.29832093943176));
#21120=CARTESIAN_POINT('Ctrl Pts',(-0.643534559198068,1.12593131807613,
2.29570408908587));
#21121=CARTESIAN_POINT('Ctrl Pts',(-0.597096971966626,1.13321234517294,
2.29308723873998));
#21122=CARTESIAN_POINT('Ctrl Pts',(-0.558034355102894,1.11949373616741,
2.29047038839408));
#21123=CARTESIAN_POINT('Ctrl Pts',(-0.518971738239162,1.10577512716188,
2.28785353804819));
#21124=CARTESIAN_POINT('Ctrl Pts',(-0.487284091743139,1.07105688205399,
2.2852366877023));
#21125=CARTESIAN_POINT('Ctrl Pts',(-0.477180536633045,1.03090707975097,
2.28261983735641));
#21126=CARTESIAN_POINT('Ctrl Pts',(-0.467076981522952,0.990757277447954,
2.28000298701051));
#21127=CARTESIAN_POINT('Ctrl Pts',(-0.478557517798788,0.945175917949804,
2.27738613666462));
#21128=CARTESIAN_POINT('Ctrl Pts',(-0.506474134662531,0.914602222071399,
2.27476928631873));
#21129=CARTESIAN_POINT('Ctrl Pts',(-0.534390751526274,0.884028526192994,
2.27215243597283));
#21130=CARTESIAN_POINT('Ctrl Pts',(-0.578743448977924,0.868462493934334,
2.26953558562694));
#21131=CARTESIAN_POINT('Ctrl Pts',(-0.6196439512168,0.874884120514905,2.26691873528105));
#21132=CARTESIAN_POINT('Ctrl Pts',(-0.660544453455676,0.881305747095476,
2.26430188493516));
#21133=CARTESIAN_POINT('Ctrl Pts',(-0.697992760481779,0.909715032515278,
2.26168503458927));
#21134=CARTESIAN_POINT('Ctrl Pts',(-0.715196605800255,0.947372914822063,
2.25906818424337));
#21135=CARTESIAN_POINT('Ctrl Pts',(-0.722669676218981,0.96373088602496,
2.2579314670416));
#21136=CARTESIAN_POINT('Ctrl Pts',(-0.72632283493267,0.981833967767914,
2.25679474983983));
#21137=CARTESIAN_POINT('Ctrl Pts',(-0.726267835011577,0.999958186565595,
2.25565803263806));
#21138=CARTESIAN_POINT('Ctrl Pts',(-0.726317906690824,1.0000827376849,2.26934196736194));
#21139=CARTESIAN_POINT('Ctrl Pts',(-0.726152658292592,0.973273988959771,
2.27102503937368));
#21140=CARTESIAN_POINT('Ctrl Pts',(-0.717783058022956,0.946370945252116,
2.27270811138542));
#21141=CARTESIAN_POINT('Ctrl Pts',(-0.701998511611248,0.924925560916646,
2.27439118339715));
#21142=CARTESIAN_POINT('Ctrl Pts',(-0.677456605234583,0.891582150162549,
2.27700803374305));
#21143=CARTESIAN_POINT('Ctrl Pts',(-0.634989648761757,0.871432202419483,
2.27962488408894));
#21144=CARTESIAN_POINT('Ctrl Pts',(-0.593640329984797,0.873511181412128,
2.28224173443483));
#21145=CARTESIAN_POINT('Ctrl Pts',(-0.552291011207836,0.875590160404774,
2.28485858478073));
#21146=CARTESIAN_POINT('Ctrl Pts',(-0.512059330126741,0.899898066133132,
2.28747543512662));
#21147=CARTESIAN_POINT('Ctrl Pts',(-0.490985651329738,0.935534969012601,
2.29009228547251));
#21148=CARTESIAN_POINT('Ctrl Pts',(-0.469911972532735,0.971171871892071,
2.2927091358184));
#21149=CARTESIAN_POINT('Ctrl Pts',(-0.467996296019824,1.01813777192265,
2.29532598616429));
#21150=CARTESIAN_POINT('Ctrl Pts',(-0.486097632801175,1.0553725535377,2.29794283651019));
#21151=CARTESIAN_POINT('Ctrl Pts',(-0.504198969582526,1.09260733515275,
2.30055968685608));
#21152=CARTESIAN_POINT('Ctrl Pts',(-0.54231731965814,1.12011099835227,2.30317653720197));
#21153=CARTESIAN_POINT('Ctrl Pts',(-0.583359963928024,1.12555066737707,
2.30579338754787));
#21154=CARTESIAN_POINT('Ctrl Pts',(-0.624402608197908,1.13099033640186,
2.30841023789376));
#21155=CARTESIAN_POINT('Ctrl Pts',(-0.668369546662063,1.11436601125193,
2.31102708823965));
#21156=CARTESIAN_POINT('Ctrl Pts',(-0.695545477203344,1.08313205274415,
2.31364393858554));
#21157=CARTESIAN_POINT('Ctrl Pts',(-0.71527010971722,1.0604620524443,2.31554328151101));
#21158=CARTESIAN_POINT('Ctrl Pts',(-0.726149173523156,1.0300956400971,2.31744262443648));
#21159=CARTESIAN_POINT('Ctrl Pts',(-0.72640212307541,0.999893075304641,
2.31934196736194));
#21160=CARTESIAN_POINT('Origin',(-0.6,1.,2.15));
#21161=CARTESIAN_POINT('',(-0.726604172280256,1.00006079745576,2.36934196736194));
#21162=CARTESIAN_POINT('',(-0.726369333664333,1.00010094057762,2.35565803263806));
#21163=CARTESIAN_POINT('',(-0.72645,1.,2.15));
#21164=CARTESIAN_POINT('',(-0.504188384727764,1.08252112989365,2.4));
#21165=CARTESIAN_POINT('Ctrl Pts',(-0.726604172280256,1.00006079745576,
2.36934196736194));
#21166=CARTESIAN_POINT('Ctrl Pts',(-0.7263677230741,0.962556440882506,2.37171076053695));
#21167=CARTESIAN_POINT('Ctrl Pts',(-0.708610935503227,0.92486733001342,
2.37407955371196));
#21168=CARTESIAN_POINT('Ctrl Pts',(-0.679417479773344,0.901356582338566,
2.37644834688697));
#21169=CARTESIAN_POINT('Ctrl Pts',(-0.647166920488327,0.875383817458018,
2.37906519723286));
#21170=CARTESIAN_POINT('Ctrl Pts',(-0.600959009984164,0.866714378341853,
2.38168204757875));
#21171=CARTESIAN_POINT('Ctrl Pts',(-0.561514903279023,0.879318622378776,
2.38429889792465));
#21172=CARTESIAN_POINT('Ctrl Pts',(-0.522070796573882,0.891922866415699,
2.38691574827054));
#21173=CARTESIAN_POINT('Ctrl Pts',(-0.489390493667762,0.92580079360571,
2.38953259861643));
#21174=CARTESIAN_POINT('Ctrl Pts',(-0.478135764397917,0.965573612020961,
2.39214944896232));
#21175=CARTESIAN_POINT('Ctrl Pts',(-0.466881035128071,1.00534643043621,
2.39476629930821));
#21176=CARTESIAN_POINT('Ctrl Pts',(-0.4770518794945,1.0510141400767,2.39738314965411));
#21177=CARTESIAN_POINT('Ctrl Pts',(-0.504188384727764,1.08252112989365,
2.4));
#21178=CARTESIAN_POINT('',(-0.695988964037237,1.08263519275223,2.4));
#21179=CARTESIAN_POINT('Origin',(-0.6,1.,2.4));
#21180=CARTESIAN_POINT('Ctrl Pts',(-0.695989827719566,1.0826357482344,2.4));
#21181=CARTESIAN_POINT('Ctrl Pts',(-0.670163685851419,1.11242103345157,
2.3975091839613));
#21182=CARTESIAN_POINT('Ctrl Pts',(-0.629259696534257,1.12936969176545,
2.3950183679226));
#21183=CARTESIAN_POINT('Ctrl Pts',(-0.589969605883147,1.12624203918417,
2.3925275518839));
#21184=CARTESIAN_POINT('Ctrl Pts',(-0.548691452172472,1.12295612861833,
2.38991070153801));
#21185=CARTESIAN_POINT('Ctrl Pts',(-0.509194654494277,1.09751079858255,
2.38729385119211));
#21186=CARTESIAN_POINT('Ctrl Pts',(-0.489166158833217,1.06128256815865,
2.38467700084622));
#21187=CARTESIAN_POINT('Ctrl Pts',(-0.469137663172157,1.02505433773475,
2.38206015050033));
#21188=CARTESIAN_POINT('Ctrl Pts',(-0.468577469528232,0.978043206922726,
2.37944330015444));
#21189=CARTESIAN_POINT('Ctrl Pts',(-0.487748907242888,0.94134646243954,
2.37682644980854));
#21190=CARTESIAN_POINT('Ctrl Pts',(-0.506920344957544,0.904649717956355,
2.37420959946265));
#21191=CARTESIAN_POINT('Ctrl Pts',(-0.54582341403078,0.878267359802006,
2.37159274911676));
#21192=CARTESIAN_POINT('Ctrl Pts',(-0.587007343519609,0.874020939484002,
2.36897589877086));
#21193=CARTESIAN_POINT('Ctrl Pts',(-0.628191273008439,0.869774519165998,
2.36635904842497));
#21194=CARTESIAN_POINT('Ctrl Pts',(-0.671656062912861,0.887664036684341,
2.36374219807908));
#21195=CARTESIAN_POINT('Ctrl Pts',(-0.697914726064929,0.919672001884272,
2.36112534773319));
#21196=CARTESIAN_POINT('Ctrl Pts',(-0.716201899123246,0.94196312902452,
2.35930290936814));
#21197=CARTESIAN_POINT('Ctrl Pts',(-0.726143981825042,0.971101800838385,
2.3574804710031));
#21198=CARTESIAN_POINT('Ctrl Pts',(-0.726369333664333,1.00010094057762,
2.35565803263806));
#21199=CARTESIAN_POINT('Origin',(0.6,1.,2.51042117235887));
#21200=CARTESIAN_POINT('',(0.44550661348391,1.00007637252271,2.03957882764113));
#21201=CARTESIAN_POINT('',(0.445941879748409,0.999994887077554,2.03542117235887));
#21202=CARTESIAN_POINT('',(0.4457,1.,2.51042117235887));
#21203=CARTESIAN_POINT('',(0.639851384185725,0.850935057178149,2.));
#21204=CARTESIAN_POINT('Ctrl Pts',(0.445941879748409,0.999994887077554,
2.03542117235887));
#21205=CARTESIAN_POINT('Ctrl Pts',(0.445958427563446,1.02606888540753,2.03408151628949));
#21206=CARTESIAN_POINT('Ctrl Pts',(0.464522119816522,1.10309173428669,2.03012500987421));
#21207=CARTESIAN_POINT('Ctrl Pts',(0.585586764715563,1.18108624726655,2.02355165311303));
#21208=CARTESIAN_POINT('Ctrl Pts',(0.74321627607811,1.11199512704675,2.01570110207536));
#21209=CARTESIAN_POINT('Ctrl Pts',(0.772174135599484,0.94213024790789,2.00785055103768));
#21210=CARTESIAN_POINT('Ctrl Pts',(0.688870364005735,0.864039910406678,
2.00261685034589));
#21211=CARTESIAN_POINT('Ctrl Pts',(0.639851384185725,0.850935057178149,
2.));
#21212=CARTESIAN_POINT('',(0.560048264277831,0.850698128346977,2.));
#21213=CARTESIAN_POINT('Origin',(0.6,1.,2.));
#21214=CARTESIAN_POINT('Ctrl Pts',(0.44550661348391,1.00007637252271,2.03957882764113));
#21215=CARTESIAN_POINT('Ctrl Pts',(0.445479076365182,1.00461168797626,2.03934410251636));
#21216=CARTESIAN_POINT('Ctrl Pts',(0.447699955244927,1.0596817411018,2.03649252704569));
#21217=CARTESIAN_POINT('Ctrl Pts',(0.513561617374857,1.15981701056446,2.03102410122914));
#21218=CARTESIAN_POINT('Ctrl Pts',(0.685634169421134,1.1602711276025,2.02317355019146));
#21219=CARTESIAN_POINT('Ctrl Pts',(0.780906782004492,1.01693885807272,2.01532299915378));
#21220=CARTESIAN_POINT('Ctrl Pts',(0.715015266367875,0.861059909554376,
2.00759848242329));
#21221=CARTESIAN_POINT('Ctrl Pts',(0.606562024823064,0.838426846369365,
2.0024908160387));
#21222=CARTESIAN_POINT('Ctrl Pts',(0.560047775926799,0.850696975355777,
2.));
#21223=CARTESIAN_POINT('Origin',(0.6,1.,2.51042117235887));
#21224=CARTESIAN_POINT('',(0.445932524475483,1.00003263872856,2.08957882764113));
#21225=CARTESIAN_POINT('',(0.445538932974414,0.999905097479817,2.08542117235887));
#21226=CARTESIAN_POINT('',(0.4457,1.,2.51042117235887));
#21227=CARTESIAN_POINT('Ctrl Pts',(0.445538932974414,0.999905097479817,
2.08542117235887));
#21228=CARTESIAN_POINT('Ctrl Pts',(0.445863620600756,1.04447123493477,2.08311595169817));
#21229=CARTESIAN_POINT('Ctrl Pts',(0.489384741719965,1.14018208017193,2.07819388069158));
#21230=CARTESIAN_POINT('Ctrl Pts',(0.651047898079357,1.17438225782416,2.0706549593391));
#21231=CARTESIAN_POINT('Ctrl Pts',(0.773614618887169,1.05360877841752,2.06280440830142));
#21232=CARTESIAN_POINT('Ctrl Pts',(0.740475677832241,0.884752178886651,
2.05495385726374));
#21233=CARTESIAN_POINT('Ctrl Pts',(0.581362560637208,0.819263360725568,
2.04710330622607));
#21234=CARTESIAN_POINT('Ctrl Pts',(0.463250898323639,0.899361552534091,
2.04059241125778));
#21235=CARTESIAN_POINT('Ctrl Pts',(0.445926103479307,0.975136595316218,
2.03669836663538));
#21236=CARTESIAN_POINT('Ctrl Pts',(0.445941879748409,0.999994887077554,
2.03542117235887));
#21237=CARTESIAN_POINT('Ctrl Pts',(0.445932524475483,1.00003263872856,2.08957882764113));
#21238=CARTESIAN_POINT('Ctrl Pts',(0.445887391771903,1.02338938965811,2.08837853792505));
#21239=CARTESIAN_POINT('Ctrl Pts',(0.461764469489331,1.09760988546538,2.08456139786307));
#21240=CARTESIAN_POINT('Ctrl Pts',(0.57612672137744,1.18012607114374,2.07812740745521));
#21241=CARTESIAN_POINT('Ctrl Pts',(0.737078048375186,1.11926881624917,2.07027685641753));
#21242=CARTESIAN_POINT('Ctrl Pts',(0.775094502137202,0.951447557128672,
2.06242630537985));
#21243=CARTESIAN_POINT('Ctrl Pts',(0.656082084236305,0.827171040068,2.05457575434217));
#21244=CARTESIAN_POINT('Ctrl Pts',(0.491836019895195,0.856969773295158,
2.04695992842926));
#21245=CARTESIAN_POINT('Ctrl Pts',(0.445786075962011,0.954049389522044,
2.04196095286225));
#21246=CARTESIAN_POINT('Ctrl Pts',(0.44550661348391,1.00007637252271,2.03957882764113));
#21247=CARTESIAN_POINT('Origin',(0.6,1.,2.51042117235887));
#21248=CARTESIAN_POINT('',(0.445609664942012,0.999879240692409,2.13957882764113));
#21249=CARTESIAN_POINT('',(0.445723577648801,1.00013290047684,2.13542117235887));
#21250=CARTESIAN_POINT('',(0.4457,1.,2.51042117235887));
#21251=CARTESIAN_POINT('Ctrl Pts',(0.445723577648801,1.00013290047684,2.13542117235887));
#21252=CARTESIAN_POINT('Ctrl Pts',(0.445613060502099,1.01281442421482,2.13476723745276));
#21253=CARTESIAN_POINT('Ctrl Pts',(0.45279637409468,1.07612012598108,2.13149645220075));
#21254=CARTESIAN_POINT('Ctrl Pts',(0.539792347657613,1.17143637275151,2.12560881660284));
#21255=CARTESIAN_POINT('Ctrl Pts',(0.70978808601476,1.14478245624706,2.11775826556517));
#21256=CARTESIAN_POINT('Ctrl Pts',(0.781323293607615,0.988284239491303,
2.10990771452749));
#21257=CARTESIAN_POINT('Ctrl Pts',(0.690243392316909,0.842292899938004,
2.10205716348982));
#21258=CARTESIAN_POINT('Ctrl Pts',(0.518231205927094,0.837737224374896,
2.09420661245213));
#21259=CARTESIAN_POINT('Ctrl Pts',(0.448527232502997,0.937309583846461,
2.08866128207516));
#21260=CARTESIAN_POINT('Ctrl Pts',(0.445495040298755,0.993880454536856,
2.08573280204407));
#21261=CARTESIAN_POINT('Ctrl Pts',(0.445538932974414,0.999905097479817,
2.08542117235887));
#21262=CARTESIAN_POINT('Ctrl Pts',(0.445609664942012,0.999879240692409,
2.13957882764113));
#21263=CARTESIAN_POINT('Ctrl Pts',(0.445970133311311,1.04180105694513,2.13741297333374));
#21264=CARTESIAN_POINT('Ctrl Pts',(0.485126633726011,1.13496755094661,2.13263026868045));
#21265=CARTESIAN_POINT('Ctrl Pts',(0.641820162707069,1.17682322770038,2.12523071368128));
#21266=CARTESIAN_POINT('Ctrl Pts',(0.770558701511974,1.06265070285456,2.11738016264359));
#21267=CARTESIAN_POINT('Ctrl Pts',(0.746336141641471,0.892291522696776,
2.10952961160592));
#21268=CARTESIAN_POINT('Ctrl Pts',(0.590875851708506,0.818527896169216,
2.10167906056824));
#21269=CARTESIAN_POINT('Ctrl Pts',(0.466115932152929,0.893907603907564,
2.09502879924665));
#21270=CARTESIAN_POINT('Ctrl Pts',(0.445985789291595,0.972467415629669,
2.09099538827094));
#21271=CARTESIAN_POINT('Ctrl Pts',(0.445932524475483,1.00003263872856,2.08957882764113));
#21272=CARTESIAN_POINT('Origin',(0.6,1.,2.51042117235887));
#21273=CARTESIAN_POINT('',(0.445644927187824,1.00012792448195,2.18957882764113));
#21274=CARTESIAN_POINT('',(0.445884646673086,0.999912830487253,2.18542117235887));
#21275=CARTESIAN_POINT('',(0.4457,1.,2.51042117235887));
#21276=CARTESIAN_POINT('Ctrl Pts',(0.445884646673086,0.999912830487253,
2.18542117235887));
#21277=CARTESIAN_POINT('Ctrl Pts',(0.446050503878428,1.03140252422683,2.18380167286145));
#21278=CARTESIAN_POINT('Ctrl Pts',(0.470644510125523,1.11401244662307,2.17956532301813));
#21279=CARTESIAN_POINT('Ctrl Pts',(0.604772735062981,1.18163868139168,2.17271212282892));
#21280=CARTESIAN_POINT('Ctrl Pts',(0.754140428515542,1.09620871962996,2.16486157179123));
#21281=CARTESIAN_POINT('Ctrl Pts',(0.765271321801097,0.924496491715462,
2.15701102075356));
#21282=CARTESIAN_POINT('Ctrl Pts',(0.628182963406343,0.820497603368372,
2.14916046971588));
#21283=CARTESIAN_POINT('Ctrl Pts',(0.479344005128078,0.872734156235485,
2.14196385358432));
#21284=CARTESIAN_POINT('Ctrl Pts',(0.446055316804476,0.962066789442876,
2.13738408779865));
#21285=CARTESIAN_POINT('Ctrl Pts',(0.445723577648801,1.00013290047684,2.13542117235887));
#21286=CARTESIAN_POINT('Ctrl Pts',(0.445644927187824,1.00012792448195,2.18957882764113));
#21287=CARTESIAN_POINT('Ctrl Pts',(0.445556744991309,1.01009369744184,2.18906425908832));
#21288=CARTESIAN_POINT('Ctrl Pts',(0.450939973182116,1.07064584055842,2.18593284018961));
#21289=CARTESIAN_POINT('Ctrl Pts',(0.530872330435983,1.16803793011858,2.18018457094502));
#21290=CARTESIAN_POINT('Ctrl Pts',(0.702033231237909,1.1503482635805,2.17233401990734));
#21291=CARTESIAN_POINT('Ctrl Pts',(0.781688304564893,0.997822700079642,
2.16448346886966));
#21292=CARTESIAN_POINT('Ctrl Pts',(0.698400986961052,0.847249790637147,
2.15663291783198));
#21293=CARTESIAN_POINT('Ctrl Pts',(0.526865324912526,0.833666900912216,
2.14878236679431));
#21294=CARTESIAN_POINT('Ctrl Pts',(0.450147764311532,0.931848543518796,
2.14309767006402));
#21295=CARTESIAN_POINT('Ctrl Pts',(0.445534604580841,0.991149857098978,
2.14002982367963));
#21296=CARTESIAN_POINT('Ctrl Pts',(0.445609664942012,0.999879240692409,
2.13957882764113));
#21297=CARTESIAN_POINT('Origin',(0.6,1.,2.51042117235887));
#21298=CARTESIAN_POINT('',(0.445922292476226,0.999948977361648,2.23957882764113));
#21299=CARTESIAN_POINT('',(0.445458679031241,0.999989078051821,2.23542117235887));
#21300=CARTESIAN_POINT('',(0.4457,1.,2.51042117235887));
#21301=CARTESIAN_POINT('Ctrl Pts',(0.445458679031242,0.999989078051821,
2.23542117235887));
#21302=CARTESIAN_POINT('Ctrl Pts',(0.445510650069037,1.04989637335789,2.23283610827014));
#21303=CARTESIAN_POINT('Ctrl Pts',(0.498659772012076,1.15041990786983,2.22763419383551));
#21304=CARTESIAN_POINT('Ctrl Pts',(0.669127678863374,1.16803795272366,2.21981542905498));
#21305=CARTESIAN_POINT('Ctrl Pts',(0.778293256865801,1.03502719068774,2.21196487801731));
#21306=CARTESIAN_POINT('Ctrl Pts',(0.727561203441069,0.870603211369231,
2.20411432697963));
#21307=CARTESIAN_POINT('Ctrl Pts',(0.562429230156179,0.822225348280642,
2.19626377594195));
#21308=CARTESIAN_POINT('Ctrl Pts',(0.458106037926808,0.910370419295299,
2.1900327244017));
#21309=CARTESIAN_POINT('Ctrl Pts',(0.445782505348105,0.980520250977966,
2.18641852320734));
#21310=CARTESIAN_POINT('Ctrl Pts',(0.445884646673086,0.999912830487253,
2.18542117235887));
#21311=CARTESIAN_POINT('Ctrl Pts',(0.445922292476226,0.999948977361648,
2.23957882764113));
#21312=CARTESIAN_POINT('Ctrl Pts',(0.446009681621634,1.02874647305155,2.23809869449701));
#21313=CARTESIAN_POINT('Ctrl Pts',(0.467487221018094,1.10857850003564,2.23400171100699));
#21314=CARTESIAN_POINT('Ctrl Pts',(0.595227265578502,1.18163865695784,2.22728787717108));
#21315=CARTESIAN_POINT('Ctrl Pts',(0.748875240939872,1.10417074102503,2.21943732613341));
#21316=CARTESIAN_POINT('Ctrl Pts',(0.769008360762544,0.933280028245809,
2.21158677509573));
#21317=CARTESIAN_POINT('Ctrl Pts',(0.637570764789711,0.822225372195567,
2.20373622405805));
#21318=CARTESIAN_POINT('Ctrl Pts',(0.483262475482066,0.867432276377129,
2.19640024157318));
#21319=CARTESIAN_POINT('Ctrl Pts',(0.446005197603095,0.959412527217309,
2.19168110943421));
#21320=CARTESIAN_POINT('Ctrl Pts',(0.445644927187824,1.00012792448195,2.18957882764113));
#21321=CARTESIAN_POINT('Origin',(0.6,1.,2.51042117235887));
#21322=CARTESIAN_POINT('',(0.445484911225394,0.999943334804163,2.28957882764113));
#21323=CARTESIAN_POINT('',(0.445861169326679,1.00010096027373,2.28542117235887));
#21324=CARTESIAN_POINT('',(0.4457,1.,2.51042117235887));
#21325=CARTESIAN_POINT('Ctrl Pts',(0.445861169326679,1.00010096027373,2.28542117235887));
#21326=CARTESIAN_POINT('Ctrl Pts',(0.445749296272184,1.01825046503264,2.28448739402472));
#21327=CARTESIAN_POINT('Ctrl Pts',(0.457041409544473,1.08712805126299,2.28093676534467));
#21328=CARTESIAN_POINT('Ctrl Pts',(0.558179831669208,1.17682325150234,2.27476928631873));
#21329=CARTESIAN_POINT('Ctrl Pts',(0.724423708785572,1.13241650393702,2.26691873528105));
#21330=CARTESIAN_POINT('Ctrl Pts',(0.779081445955335,0.969255483615749,
2.25906818424337));
#21331=CARTESIAN_POINT('Ctrl Pts',(0.673134684925636,0.833666878534013,
2.25121763320569));
#21332=CARTESIAN_POINT('Ctrl Pts',(0.50159899980171,0.84724977008965,2.24336708216802));
#21333=CARTESIAN_POINT('Ctrl Pts',(0.445736890155226,0.948241381044753,
2.23810159521908));
#21334=CARTESIAN_POINT('Ctrl Pts',(0.445458039989146,0.999375411980858,
2.23545295861603));
#21335=CARTESIAN_POINT('Ctrl Pts',(0.445458679031242,0.999989078051821,
2.23542117235887));
#21336=CARTESIAN_POINT('Ctrl Pts',(0.445484911225394,0.999943334804162,
2.28957882764113));
#21337=CARTESIAN_POINT('Ctrl Pts',(0.445711121771824,1.04718147797272,2.2871331299057));
#21338=CARTESIAN_POINT('Ctrl Pts',(0.493918064875951,1.14536352796849,2.28207058182437));
#21339=CARTESIAN_POINT('Ctrl Pts',(0.660207644220989,1.17143634973614,2.27439118339715));
#21340=CARTESIAN_POINT('Ctrl Pts',(0.776207730757634,1.04434204382826,2.26654063235948));
#21341=CARTESIAN_POINT('Ctrl Pts',(0.734180526190243,0.87748075149375,2.2586900813218));
#21342=CARTESIAN_POINT('Ctrl Pts',(0.571817040388558,0.820497627508739,
2.25083953028412));
#21343=CARTESIAN_POINT('Ctrl Pts',(0.460575165814633,0.904888683245033,
2.24446911239056));
#21344=CARTESIAN_POINT('Ctrl Pts',(0.445855179091712,0.977832988101724,
2.2407155448429));
#21345=CARTESIAN_POINT('Ctrl Pts',(0.445922292476226,0.999948977361648,
2.23957882764113));
#21346=CARTESIAN_POINT('Origin',(0.6,1.,2.51042117235887));
#21347=CARTESIAN_POINT('',(0.445798439227784,1.00012317213786,2.33957882764113));
#21348=CARTESIAN_POINT('',(0.445758404806891,0.999869526120069,2.33542117235887));
#21349=CARTESIAN_POINT('',(0.4457,1.,2.51042117235887));
#21350=CARTESIAN_POINT('Ctrl Pts',(0.445758404806891,0.999869526120069,
2.33542117235887));
#21351=CARTESIAN_POINT('Ctrl Pts',(0.446067065282869,1.03672406343128,2.33352182943341));
#21352=CARTESIAN_POINT('Ctrl Pts',(0.477632210806756,1.12483092984331,2.32900563616205));
#21353=CARTESIAN_POINT('Ctrl Pts',(0.623873281963166,1.1801260959606,2.3218725925448));
#21354=CARTESIAN_POINT('Ctrl Pts',(0.76341449322476,1.07944244879737,2.31402204150712));
#21355=CARTESIAN_POINT('Ctrl Pts',(0.756401707578768,0.907512694301026,
2.30617149046944));
#21356=CARTESIAN_POINT('Ctrl Pts',(0.609124149502328,0.818527871661859,
2.29832093943176));
#21357=CARTESIAN_POINT('Ctrl Pts',(0.472154957249585,0.883517743796439,
2.29140416672824));
#21358=CARTESIAN_POINT('Ctrl Pts',(0.446062812907388,0.967387710919709,
2.28710424437061));
#21359=CARTESIAN_POINT('Ctrl Pts',(0.445861169326679,1.00010096027373,2.28542117235887));
#21360=CARTESIAN_POINT('Ctrl Pts',(0.445798439227784,1.00012317213786,2.33957882764113));
#21361=CARTESIAN_POINT('Ctrl Pts',(0.445678571748812,1.01554817070058,2.33878441566028));
#21362=CARTESIAN_POINT('Ctrl Pts',(0.454838216821075,1.08164530296445,2.33537315333353));
#21363=CARTESIAN_POINT('Ctrl Pts',(0.548952109888326,1.17438223097154,2.3293450406609));
#21364=CARTESIAN_POINT('Ctrl Pts',(0.717297767916034,1.1387683610531,2.32149448962322));
#21365=CARTESIAN_POINT('Ctrl Pts',(0.780449022522885,0.978702297157564,
2.31364393858554));
#21366=CARTESIAN_POINT('Ctrl Pts',(0.681768782849741,0.837737246759644,
2.30579338754786));
#21367=CARTESIAN_POINT('Ctrl Pts',(0.509756619949943,0.842292920851884,
2.29794283651019));
#21368=CARTESIAN_POINT('Ctrl Pts',(0.447051029253845,0.942803275635825,
2.29253798320794));
#21369=CARTESIAN_POINT('Ctrl Pts',(0.445469080763202,0.996637557724894,
2.28974998025159));
#21370=CARTESIAN_POINT('Ctrl Pts',(0.445484911225394,0.999943334804162,
2.28957882764113));
#21371=CARTESIAN_POINT('Origin',(0.6,1.,2.51042117235887));
#21372=CARTESIAN_POINT('',(0.445864724392684,0.99983533609866,2.38957882764113));
#21373=CARTESIAN_POINT('',(0.44551185913013,1.0000741974826,2.38542117235887));
#21374=CARTESIAN_POINT('',(0.4457,1.,2.51042117235887));
#21375=CARTESIAN_POINT('',(0.560148615814278,0.850935057178148,2.4));
#21376=CARTESIAN_POINT('Ctrl Pts',(0.560148615814278,0.850935057178148,
2.4));
#21377=CARTESIAN_POINT('Ctrl Pts',(0.511129635994267,0.864039910406677,
2.39738314965411));
#21378=CARTESIAN_POINT('Ctrl Pts',(0.455839024989005,0.915869990257929,
2.39390942553448));
#21379=CARTESIAN_POINT('Ctrl Pts',(0.445750544275333,0.983186184474914,
2.39043570141486));
#21380=CARTESIAN_POINT('Ctrl Pts',(0.445864724392684,0.99983533609866,2.38957882764113));
#21381=CARTESIAN_POINT('',(0.639951772688379,0.850698147244252,2.4));
#21382=CARTESIAN_POINT('Origin',(0.6,1.,2.4));
#21383=CARTESIAN_POINT('Ctrl Pts',(0.639952262351544,0.850696991672977,
2.4));
#21384=CARTESIAN_POINT('Ctrl Pts',(0.593438030028895,0.838426877605595,
2.3975091839613));
#21385=CARTESIAN_POINT('Ctrl Pts',(0.490251767896999,0.859960628309645,
2.39264957474759));
#21386=CARTESIAN_POINT('Ctrl Pts',(0.445800376826071,0.954309672447724,
2.38778996553388));
#21387=CARTESIAN_POINT('Ctrl Pts',(0.445511859130131,1.0000741974826,2.38542117235887));
#21388=CARTESIAN_POINT('Origin',(-0.6,1.,2.51042117235887));
#21389=CARTESIAN_POINT('',(-0.75449339269049,1.00007637145626,2.03957882764113));
#21390=CARTESIAN_POINT('',(-0.754058103775977,0.999994895029031,2.03542117235887));
#21391=CARTESIAN_POINT('',(-0.7543,1.,2.51042117235887));
#21392=CARTESIAN_POINT('',(-0.560148615814275,0.850935057178149,2.));
#21393=CARTESIAN_POINT('Ctrl Pts',(-0.754058103775977,0.999994895029031,
2.03542117235887));
#21394=CARTESIAN_POINT('Ctrl Pts',(-0.754041555268885,1.02606889659328,
2.03408151628949));
#21395=CARTESIAN_POINT('Ctrl Pts',(-0.735477862467914,1.10309174989979,
2.03012500987421));
#21396=CARTESIAN_POINT('Ctrl Pts',(-0.614413230072635,1.18108614472194,
2.02355165311304));
#21397=CARTESIAN_POINT('Ctrl Pts',(-0.456783762484268,1.11199525865091,
2.01570110207535));
#21398=CARTESIAN_POINT('Ctrl Pts',(-0.427825820216639,0.942129974923708,
2.00785055103768));
#21399=CARTESIAN_POINT('Ctrl Pts',(-0.511129635994264,0.864039910406679,
2.00261685034589));
#21400=CARTESIAN_POINT('Ctrl Pts',(-0.560148615814275,0.850935057178149,
2.));
#21401=CARTESIAN_POINT('',(-0.639951747396791,0.850698134330425,2.));
#21402=CARTESIAN_POINT('Origin',(-0.6,1.,2.));
#21403=CARTESIAN_POINT('Ctrl Pts',(-0.754493392690491,1.00007637145626,
2.03957882764113));
#21404=CARTESIAN_POINT('Ctrl Pts',(-0.754520929823858,1.00461168712382,
2.03934410251636));
#21405=CARTESIAN_POINT('Ctrl Pts',(-0.752300051092223,1.05968174304917,
2.03649252704569));
#21406=CARTESIAN_POINT('Ctrl Pts',(-0.686438388751686,1.15981702310584,
2.03102410122914));
#21407=CARTESIAN_POINT('Ctrl Pts',(-0.514365822072695,1.16027112465931,
2.02317355019146));
#21408=CARTESIAN_POINT('Ctrl Pts',(-0.41909321999119,1.01693887482571,2.01532299915378));
#21409=CARTESIAN_POINT('Ctrl Pts',(-0.484984709990756,0.861059878644944,
2.00759848242329));
#21410=CARTESIAN_POINT('Ctrl Pts',(-0.593437992489385,0.838426856238601,
2.0024908160387));
#21411=CARTESIAN_POINT('Ctrl Pts',(-0.63995223616215,0.850696980524376,
2.));
#21412=CARTESIAN_POINT('Origin',(-0.6,1.,2.51042117235887));
#21413=CARTESIAN_POINT('',(-0.754067482051008,1.00003263870824,2.08957882764113));
#21414=CARTESIAN_POINT('',(-0.754461050156182,0.999905097350985,2.08542117235887));
#21415=CARTESIAN_POINT('',(-0.7543,1.,2.51042117235887));
#21416=CARTESIAN_POINT('Ctrl Pts',(-0.754461050156182,0.999905097350985,
2.08542117235887));
#21417=CARTESIAN_POINT('Ctrl Pts',(-0.754136362473472,1.0444712301837,2.08311595169818));
#21418=CARTESIAN_POINT('Ctrl Pts',(-0.71061524567478,1.14018206615738,2.07819388069158));
#21419=CARTESIAN_POINT('Ctrl Pts',(-0.548952108412014,1.17438223594748,
2.0706549593391));
#21420=CARTESIAN_POINT('Ctrl Pts',(-0.426385398697532,1.05360877753029,
2.06280440830142));
#21421=CARTESIAN_POINT('Ctrl Pts',(-0.459524339782119,0.884752182582313,
2.05495385726375));
#21422=CARTESIAN_POINT('Ctrl Pts',(-0.618637434184013,0.819263396393857,
2.04710330622607));
#21423=CARTESIAN_POINT('Ctrl Pts',(-0.736749089275893,0.89936154319225,
2.04059241125778));
#21424=CARTESIAN_POINT('Ctrl Pts',(-0.754073880704865,0.975136600184218,
2.03669836663538));
#21425=CARTESIAN_POINT('Ctrl Pts',(-0.754058103775977,0.999994895029031,
2.03542117235887));
#21426=CARTESIAN_POINT('Ctrl Pts',(-0.754067482051008,1.00003263870824,
2.08957882764113));
#21427=CARTESIAN_POINT('Ctrl Pts',(-0.754112614754579,1.02338939061779,
2.08837853792505));
#21428=CARTESIAN_POINT('Ctrl Pts',(-0.738235536361179,1.09760988955354,
2.08456139786307));
#21429=CARTESIAN_POINT('Ctrl Pts',(-0.623873279675432,1.18012607896462,
2.0781274074552));
#21430=CARTESIAN_POINT('Ctrl Pts',(-0.462921945732953,1.11926882096942,
2.07027685641753));
#21431=CARTESIAN_POINT('Ctrl Pts',(-0.424905490600427,0.951447555675582,
2.06242630537985));
#21432=CARTESIAN_POINT('Ctrl Pts',(-0.54391791306908,0.827171031659744,
2.05457575434217));
#21433=CARTESIAN_POINT('Ctrl Pts',(-0.708163985289881,0.856969769057042,
2.04695992842926));
#21434=CARTESIAN_POINT('Ctrl Pts',(-0.754213930063824,0.954049386283767,
2.04196095286225));
#21435=CARTESIAN_POINT('Ctrl Pts',(-0.754493392690491,1.00007637145626,
2.03957882764113));
#21436=CARTESIAN_POINT('Origin',(-0.6,1.,2.51042117235887));
#21437=CARTESIAN_POINT('',(-0.754390341602871,0.999879240687419,2.13957882764113));
#21438=CARTESIAN_POINT('',(-0.75427640544451,1.00013290045585,2.13542117235887));
#21439=CARTESIAN_POINT('',(-0.7543,1.,2.51042117235887));
#21440=CARTESIAN_POINT('Ctrl Pts',(-0.75427640544451,1.00013290045585,2.13542117235887));
#21441=CARTESIAN_POINT('Ctrl Pts',(-0.754386922579298,1.01281442280347,
2.13476723745276));
#21442=CARTESIAN_POINT('Ctrl Pts',(-0.747203609773684,1.07612011763199,
2.13149645220075));
#21443=CARTESIAN_POINT('Ctrl Pts',(-0.660207645725328,1.17143635399922,
2.12560881660285));
#21444=CARTESIAN_POINT('Ctrl Pts',(-0.490211926051119,1.14478244030651,
2.11775826556517));
#21445=CARTESIAN_POINT('Ctrl Pts',(-0.418676726208604,0.988284240908056,
2.10990771452749));
#21446=CARTESIAN_POINT('Ctrl Pts',(-0.509756617677689,0.842292916978238,
2.10205716348981));
#21447=CARTESIAN_POINT('Ctrl Pts',(-0.681768784928714,0.837737242612945,
2.09420661245213));
#21448=CARTESIAN_POINT('Ctrl Pts',(-0.75147275106401,0.937309590263154,
2.08866128207516));
#21449=CARTESIAN_POINT('Ctrl Pts',(-0.754504942839462,0.993880455032877,
2.08573280204407));
#21450=CARTESIAN_POINT('Ctrl Pts',(-0.754461050156182,0.999905097350985,
2.08542117235887));
#21451=CARTESIAN_POINT('Ctrl Pts',(-0.75439034160287,0.999879240687419,
2.13957882764113));
#21452=CARTESIAN_POINT('Ctrl Pts',(-0.754029873218229,1.04180105871682,
2.13741297333374));
#21453=CARTESIAN_POINT('Ctrl Pts',(-0.714873371143386,1.13496755666601,
2.13263026868045));
#21454=CARTESIAN_POINT('Ctrl Pts',(-0.558179835520779,1.17682323520091,
2.12523071368127));
#21455=CARTESIAN_POINT('Ctrl Pts',(-0.429441291256411,1.0626507055017,2.1173801626436));
#21456=CARTESIAN_POINT('Ctrl Pts',(-0.453663852157743,0.892291518147041,
2.10952961160592));
#21457=CARTESIAN_POINT('Ctrl Pts',(-0.609124148673025,0.818527888446316,
2.10167906056824));
#21458=CARTESIAN_POINT('Ctrl Pts',(-0.733884073530661,0.893907599452349,
2.09502879924664));
#21459=CARTESIAN_POINT('Ctrl Pts',(-0.754014217234906,0.972467414452767,
2.09099538827094));
#21460=CARTESIAN_POINT('Ctrl Pts',(-0.754067482051008,1.00003263870824,
2.08957882764113));
#21461=CARTESIAN_POINT('Origin',(-0.6,1.,2.51042117235887));
#21462=CARTESIAN_POINT('',(-0.754355079355554,1.00012792448738,2.18957882764113));
#21463=CARTESIAN_POINT('',(-0.754115336434833,0.999912830496762,2.18542117235887));
#21464=CARTESIAN_POINT('',(-0.7543,1.,2.51042117235887));
#21465=CARTESIAN_POINT('Ctrl Pts',(-0.754115336434833,0.999912830496762,
2.18542117235887));
#21466=CARTESIAN_POINT('Ctrl Pts',(-0.753949479247709,1.03140252078477,
2.18380167286145));
#21467=CARTESIAN_POINT('Ctrl Pts',(-0.72935547569638,1.11401243412622,2.17956532301813));
#21468=CARTESIAN_POINT('Ctrl Pts',(-0.595227265459685,1.1816386614837,2.17271212282892));
#21469=CARTESIAN_POINT('Ctrl Pts',(-0.445859588380167,1.09620870908317,
2.16486157179124));
#21470=CARTESIAN_POINT('Ctrl Pts',(-0.434728696312199,0.924496499994273,
2.15701102075356));
#21471=CARTESIAN_POINT('Ctrl Pts',(-0.571817039685625,0.820497623037239,
2.14916046971588));
#21472=CARTESIAN_POINT('Ctrl Pts',(-0.720655981642513,0.872734170194251,
2.14196385358432));
#21473=CARTESIAN_POINT('Ctrl Pts',(-0.753944666324598,0.962066793595335,
2.13738408779865));
#21474=CARTESIAN_POINT('Ctrl Pts',(-0.75427640544451,1.00013290045585,2.13542117235887));
#21475=CARTESIAN_POINT('Ctrl Pts',(-0.754355079355553,1.00012792448738,
2.18957882764113));
#21476=CARTESIAN_POINT('Ctrl Pts',(-0.754443261555807,1.01009369786974,
2.18906425908832));
#21477=CARTESIAN_POINT('Ctrl Pts',(-0.749060033136799,1.07064584355324,
2.18593284018961));
#21478=CARTESIAN_POINT('Ctrl Pts',(-0.669127672494447,1.16803793724193,
2.18018457094502));
#21479=CARTESIAN_POINT('Ctrl Pts',(-0.497966764436741,1.15034826995414,
2.17233401990734));
#21480=CARTESIAN_POINT('Ctrl Pts',(-0.418311687733005,0.997822699987136,
2.16448346886966));
#21481=CARTESIAN_POINT('Ctrl Pts',(-0.501599008867606,0.847249784162188,
2.15663291783199));
#21482=CARTESIAN_POINT('Ctrl Pts',(-0.673134678187691,0.833666893860354,
2.1487823667943));
#21483=CARTESIAN_POINT('Ctrl Pts',(-0.749852242041061,0.931848540630513,
2.14309767006402));
#21484=CARTESIAN_POINT('Ctrl Pts',(-0.754465401967237,0.99114985672403,
2.14002982367963));
#21485=CARTESIAN_POINT('Ctrl Pts',(-0.75439034160287,0.999879240687419,
2.13957882764113));
#21486=CARTESIAN_POINT('Origin',(-0.6,1.,2.51042117235887));
#21487=CARTESIAN_POINT('',(-0.75407771405525,0.999948977359204,2.23957882764113));
#21488=CARTESIAN_POINT('',(-0.754541304029948,0.999989078053162,2.23542117235887));
#21489=CARTESIAN_POINT('',(-0.7543,1.,2.51042117235887));
#21490=CARTESIAN_POINT('Ctrl Pts',(-0.754541304029948,0.999989078053162,
2.23542117235887));
#21491=CARTESIAN_POINT('Ctrl Pts',(-0.754489332997837,1.04989636788915,
2.23283610827014));
#21492=CARTESIAN_POINT('Ctrl Pts',(-0.701340216880369,1.15041989138249,
2.2276341938355));
#21493=CARTESIAN_POINT('Ctrl Pts',(-0.530872328713473,1.16803793430571,
2.21981542905499));
#21494=CARTESIAN_POINT('Ctrl Pts',(-0.421706762676398,1.0350271868484,2.2119648780173));
#21495=CARTESIAN_POINT('Ctrl Pts',(-0.472438810540477,0.870603225552124,
2.20411432697963));
#21496=CARTESIAN_POINT('Ctrl Pts',(-0.637570765725878,0.822225367765818,
2.19626377594195));
#21497=CARTESIAN_POINT('Ctrl Pts',(-0.741893946520544,0.910370429119493,
2.1900327244017));
#21498=CARTESIAN_POINT('Ctrl Pts',(-0.754217477748594,0.980520253113081,
2.18641852320734));
#21499=CARTESIAN_POINT('Ctrl Pts',(-0.754115336434833,0.999912830496762,
2.18542117235887));
#21500=CARTESIAN_POINT('Ctrl Pts',(-0.75407771405525,0.999948977359204,
2.23957882764113));
#21501=CARTESIAN_POINT('Ctrl Pts',(-0.753990324906209,1.02874647427002,
2.23809869449701));
#21502=CARTESIAN_POINT('Ctrl Pts',(-0.732512784599607,1.10857850463897,
2.23400171100699));
#21503=CARTESIAN_POINT('Ctrl Pts',(-0.604772734623643,1.18163866465747,
2.22728787717109));
#21504=CARTESIAN_POINT('Ctrl Pts',(-0.451124752749149,1.10417074544119,
2.21943732613341));
#21505=CARTESIAN_POINT('Ctrl Pts',(-0.43099163207285,0.933280025417337,
2.21158677509573));
#21506=CARTESIAN_POINT('Ctrl Pts',(-0.562429233617627,0.822225364659454,
2.20373622405805));
#21507=CARTESIAN_POINT('Ctrl Pts',(-0.716737529466624,0.867432270757321,
2.19640024157319));
#21508=CARTESIAN_POINT('Ctrl Pts',(-0.753994808925007,0.959412525496741,
2.19168110943421));
#21509=CARTESIAN_POINT('Ctrl Pts',(-0.754355079355553,1.00012792448738,
2.18957882764113));
#21510=CARTESIAN_POINT('Origin',(-0.6,1.,2.51042117235887));
#21511=CARTESIAN_POINT('',(-0.754515095317817,0.999943334786189,2.28957882764113));
#21512=CARTESIAN_POINT('',(-0.754138813779314,1.00010096025924,2.28542117235887));
#21513=CARTESIAN_POINT('',(-0.7543,1.,2.51042117235887));
#21514=CARTESIAN_POINT('Ctrl Pts',(-0.754138813779314,1.00010096025924,
2.28542117235887));
#21515=CARTESIAN_POINT('Ctrl Pts',(-0.754250686820938,1.01825046303266,
2.28448739402472));
#21516=CARTESIAN_POINT('Ctrl Pts',(-0.74295857478395,1.08712804172823,2.28093676534467));
#21517=CARTESIAN_POINT('Ctrl Pts',(-0.641820163748749,1.17682323210921,
2.27476928631873));
#21518=CARTESIAN_POINT('Ctrl Pts',(-0.47557630485125,1.13241648942973,2.26691873528105));
#21519=CARTESIAN_POINT('Ctrl Pts',(-0.420918573673669,0.969255486982105,
2.25906818424337));
#21520=CARTESIAN_POINT('Ctrl Pts',(-0.526865323090207,0.833666896767115,
2.2512176332057));
#21521=CARTESIAN_POINT('Ctrl Pts',(-0.698400989412974,0.847249786831145,
2.24336708216802));
#21522=CARTESIAN_POINT('Ctrl Pts',(-0.75426309293647,0.948241386717884,
2.23810159521908));
#21523=CARTESIAN_POINT('Ctrl Pts',(-0.754541943071973,0.999375412049459,
2.23545295861603));
#21524=CARTESIAN_POINT('Ctrl Pts',(-0.754541304029948,0.999989078053162,
2.23542117235887));
#21525=CARTESIAN_POINT('Ctrl Pts',(-0.754515095317817,0.999943334786189,
2.28957882764113));
#21526=CARTESIAN_POINT('Ctrl Pts',(-0.754288884759399,1.04718147995109,
2.2871331299057));
#21527=CARTESIAN_POINT('Ctrl Pts',(-0.706081939633174,1.1453635341575,2.28207058182437));
#21528=CARTESIAN_POINT('Ctrl Pts',(-0.539792353219763,1.17143635698873,
2.27439118339715));
#21529=CARTESIAN_POINT('Ctrl Pts',(-0.423792261776434,1.04434204571596,
2.26654063235948));
#21530=CARTESIAN_POINT('Ctrl Pts',(-0.465819468119529,0.877480746295693,
2.2586900813218));
#21531=CARTESIAN_POINT('Ctrl Pts',(-0.6281829608073,0.820497619901593,2.25083953028412));
#21532=CARTESIAN_POINT('Ctrl Pts',(-0.73942484009554,0.90488867921255,2.24446911239056));
#21533=CARTESIAN_POINT('Ctrl Pts',(-0.754144827442555,0.977832987161639,
2.2407155448429));
#21534=CARTESIAN_POINT('Ctrl Pts',(-0.75407771405525,0.999948977359204,
2.23957882764113));
#21535=CARTESIAN_POINT('Origin',(-0.6,1.,2.51042117235887));
#21536=CARTESIAN_POINT('',(-0.754201567294635,1.0001231722509,2.33957882764113));
#21537=CARTESIAN_POINT('',(-0.754241578414675,0.999869525658411,2.33542117235887));
#21538=CARTESIAN_POINT('',(-0.7543,1.,2.51042117235887));
#21539=CARTESIAN_POINT('Ctrl Pts',(-0.754241578414675,0.999869525658411,
2.33542117235887));
#21540=CARTESIAN_POINT('Ctrl Pts',(-0.753932917948777,1.03672405905087,
2.33352182943341));
#21541=CARTESIAN_POINT('Ctrl Pts',(-0.72236777560142,1.12483091690338,2.32900563616205));
#21542=CARTESIAN_POINT('Ctrl Pts',(-0.576126720758545,1.18012607574093,
2.3218725925448));
#21543=CARTESIAN_POINT('Ctrl Pts',(-0.436585524633584,1.079442440351,2.31402204150712));
#21544=CARTESIAN_POINT('Ctrl Pts',(-0.443598309590693,0.907512704295987,
2.30617149046944));
#21545=CARTESIAN_POINT('Ctrl Pts',(-0.59087585148424,0.818527891629664,
2.29832093943176));
#21546=CARTESIAN_POINT('Ctrl Pts',(-0.727845028742113,0.883517756536112,
2.29140416672824));
#21547=CARTESIAN_POINT('Ctrl Pts',(-0.753937170221803,0.967387714483928,
2.28710424437061));
#21548=CARTESIAN_POINT('Ctrl Pts',(-0.754138813779314,1.00010096025924,
2.28542117235887));
#21549=CARTESIAN_POINT('Ctrl Pts',(-0.754201567294635,1.0001231722509,2.33957882764113));
#21550=CARTESIAN_POINT('Ctrl Pts',(-0.754321434708458,1.01554817119723,
2.33878441566028));
#21551=CARTESIAN_POINT('Ctrl Pts',(-0.745161788983251,1.08164530518807,
2.33537315333353));
#21552=CARTESIAN_POINT('Ctrl Pts',(-0.651047892623131,1.17438223943631,
2.3293450406609));
#21553=CARTESIAN_POINT('Ctrl Pts',(-0.48270222690289,1.13876836634555,2.32149448962322));
#21554=CARTESIAN_POINT('Ctrl Pts',(-0.419550969949932,0.978702296577685,
2.31364393858554));
#21555=CARTESIAN_POINT('Ctrl Pts',(-0.518231213613428,0.837737239705173,
2.30579338754787));
#21556=CARTESIAN_POINT('Ctrl Pts',(-0.690243383915708,0.842292914261777,
2.29794283651019));
#21557=CARTESIAN_POINT('Ctrl Pts',(-0.752948977226896,0.9428032732054,2.29253798320794));
#21558=CARTESIAN_POINT('Ctrl Pts',(-0.754530925780848,0.996637557567215,
2.28974998025159));
#21559=CARTESIAN_POINT('Ctrl Pts',(-0.754515095317817,0.999943334786189,
2.28957882764113));
#21560=CARTESIAN_POINT('Origin',(-0.6,1.,2.51042117235887));
#21561=CARTESIAN_POINT('',(-0.754135271629158,0.999835375941562,2.38957882764113));
#21562=CARTESIAN_POINT('',(-0.754488127978201,1.0000741878009,2.38542117235887));
#21563=CARTESIAN_POINT('',(-0.7543,1.,2.51042117235887));
#21564=CARTESIAN_POINT('',(-0.639851384185722,0.850935057178148,2.4));
#21565=CARTESIAN_POINT('Ctrl Pts',(-0.639851384185722,0.850935057178148,
2.4));
#21566=CARTESIAN_POINT('Ctrl Pts',(-0.688870364005733,0.864039910406677,
2.39738314965411));
#21567=CARTESIAN_POINT('Ctrl Pts',(-0.744160963654378,0.915870060408085,
2.39390942553448));
#21568=CARTESIAN_POINT('Ctrl Pts',(-0.754249449960209,0.983186232192211,
2.39043570141486));
#21569=CARTESIAN_POINT('Ctrl Pts',(-0.754135271629158,0.999835375941562,
2.38957882764113));
#21570=CARTESIAN_POINT('',(-0.560048257412569,0.850698131867252,2.4));
#21571=CARTESIAN_POINT('Origin',(-0.6,1.,2.4));
#21572=CARTESIAN_POINT('Ctrl Pts',(-0.56004776881791,0.850696978396875,
2.4));
#21573=CARTESIAN_POINT('Ctrl Pts',(-0.606562014643699,0.838426852173434,
2.3975091839613));
#21574=CARTESIAN_POINT('Ctrl Pts',(-0.709748176229453,0.859960702974294,
2.39264957474759));
#21575=CARTESIAN_POINT('Ctrl Pts',(-0.754199601979702,0.954309678356425,
2.38778996553388));
#21576=CARTESIAN_POINT('Ctrl Pts',(-0.754488127978201,1.0000741878009,2.38542117235887));
#21577=CARTESIAN_POINT('Origin',(-0.6,1.,2.51042117235887));
#21578=CARTESIAN_POINT('Ctrl Pts',(-0.754488127978201,1.0000741878009,2.38542117235887));
#21579=CARTESIAN_POINT('Ctrl Pts',(-0.754518342073576,1.00486659216084,
2.38517311518799));
#21580=CARTESIAN_POINT('Ctrl Pts',(-0.75215961407118,1.06018735745674,2.38230820767121));
#21581=CARTESIAN_POINT('Ctrl Pts',(-0.685634174422424,1.16027112587027,
2.37682644980854));
#21582=CARTESIAN_POINT('Ctrl Pts',(-0.513561613772921,1.15981701793772,
2.36897589877087));
#21583=CARTESIAN_POINT('Ctrl Pts',(-0.419009660745144,1.01606137072615,
2.36112534773318));
#21584=CARTESIAN_POINT('Ctrl Pts',(-0.486773837186857,0.857888188850051,
2.35327479669551));
#21585=CARTESIAN_POINT('Ctrl Pts',(-0.656082085820325,0.827171035125292,
2.34542424565783));
#21586=CARTESIAN_POINT('Ctrl Pts',(-0.746300935356365,0.921380401738197,
2.33947303754562));
#21587=CARTESIAN_POINT('Ctrl Pts',(-0.754358179883375,0.985947131323567,
2.3361386797793));
#21588=CARTESIAN_POINT('Ctrl Pts',(-0.754241578414675,0.999869525658411,
2.33542117235887));
#21589=CARTESIAN_POINT('Ctrl Pts',(-0.754135271629158,0.999835375941562,
2.38957882764113));
#21590=CARTESIAN_POINT('Ctrl Pts',(-0.753900754954872,1.03403189804748,
2.38781885106897));
#21591=CARTESIAN_POINT('Ctrl Pts',(-0.726011265053425,1.1195363898437,2.38344202415091));
#21592=CARTESIAN_POINT('Ctrl Pts',(-0.585586769094172,1.18108616109394,
2.37644834688697));
#21593=CARTESIAN_POINT('Ctrl Pts',(-0.44099944093888,1.08793753892263,2.36859779584929));
#21594=CARTESIAN_POINT('Ctrl Pts',(-0.438948720197302,0.915842224941729,
2.36074724481161));
#21595=CARTESIAN_POINT('Ctrl Pts',(-0.581362564989717,0.819263390701727,
2.35289669377393));
#21596=CARTESIAN_POINT('Ctrl Pts',(-0.724374710267433,0.878125248400964,
2.34584055471711));
#21597=CARTESIAN_POINT('Ctrl Pts',(-0.753926582804302,0.964737112450477,
2.34140126600617));
#21598=CARTESIAN_POINT('Ctrl Pts',(-0.754201567294635,1.0001231722509,2.33957882764113));
#21599=CARTESIAN_POINT('Ctrl Pts',(-0.504188384727764,1.08252112989365,
2.4));
#21600=CARTESIAN_POINT('Ctrl Pts',(-0.4770518794945,1.0510141400767,2.39738314965411));
#21601=CARTESIAN_POINT('Ctrl Pts',(-0.456710190761643,0.959678720795721,
2.39214944896232));
#21602=CARTESIAN_POINT('Ctrl Pts',(-0.554751099480001,0.858044939225688,
2.38429889792465));
#21603=CARTESIAN_POINT('Ctrl Pts',(-0.69337483099249,0.884053256574183,
2.37644834688697));
#21604=CARTESIAN_POINT('Ctrl Pts',(-0.7482544551901,1.01388152850897,2.36859779584929));
#21605=CARTESIAN_POINT('Ctrl Pts',(-0.670177844171844,1.13134338215356,
2.36074724481161));
#21606=CARTESIAN_POINT('Ctrl Pts',(-0.52916309826044,1.13097123731837,2.35289669377393));
#21607=CARTESIAN_POINT('Ctrl Pts',(-0.451677068057184,1.01316241301569,
2.34504614273626));
#21608=CARTESIAN_POINT('Ctrl Pts',(-0.507210315698497,0.883538311601356,
2.33719559169857));
#21609=CARTESIAN_POINT('Ctrl Pts',(-0.645959687310304,0.858365375188547,
2.3293450406609));
#21610=CARTESIAN_POINT('Ctrl Pts',(-0.743491252981436,0.960210910505111,
2.32149448962322));
#21611=CARTESIAN_POINT('Ctrl Pts',(-0.712336485126218,1.097741686102,2.31364393858554));
#21612=CARTESIAN_POINT('Ctrl Pts',(-0.580435669733753,1.14761466155179,
2.30579338754787));
#21613=CARTESIAN_POINT('Ctrl Pts',(-0.466080619506913,1.06510367195323,
2.29794283651019));
#21614=CARTESIAN_POINT('Ctrl Pts',(-0.471827649045646,0.924205971861489,
2.29009228547251));
#21615=CARTESIAN_POINT('Ctrl Pts',(-0.592522692288931,0.851282254676416,
2.28224173443483));
#21616=CARTESIAN_POINT('Ctrl Pts',(-0.719923561707409,0.911732097905615,
2.27439118339715));
#21617=CARTESIAN_POINT('Ctrl Pts',(-0.739774130548921,1.051342719201,2.26654063235948));
#21618=CARTESIAN_POINT('Ctrl Pts',(-0.634271935878349,1.14490795657946,
2.2586900813218));
#21619=CARTESIAN_POINT('Ctrl Pts',(-0.498033854494106,1.10851629998956,
2.25083953028412));
#21620=CARTESIAN_POINT('Ctrl Pts',(-0.453241436429265,0.974804642442561,
2.24298897924644));
#21621=CARTESIAN_POINT('Ctrl Pts',(-0.540065587198681,0.86368878221777,
2.23513842820877));
#21622=CARTESIAN_POINT('Ctrl Pts',(-0.680640344207846,0.874820061858706,
2.22728787717108));
#21623=CARTESIAN_POINT('Ctrl Pts',(-0.748894923426505,0.998215686443256,
2.21943732613341));
#21624=CARTESIAN_POINT('Ctrl Pts',(-0.68361699553809,1.12321152562211,2.21158677509573));
#21625=CARTESIAN_POINT('Ctrl Pts',(-0.543349358171216,1.13770833955254,
2.20373622405805));
#21626=CARTESIAN_POINT('Ctrl Pts',(-0.453887363191384,1.02870504068037,
2.19588567302037));
#21627=CARTESIAN_POINT('Ctrl Pts',(-0.49546265452264,0.893958378944044,
2.1880351219827));
#21628=CARTESIAN_POINT('Ctrl Pts',(-0.630789522527785,0.854312363927335,
2.18018457094502));
#21629=CARTESIAN_POINT('Ctrl Pts',(-0.73850361471777,0.945322484520081,
2.17233401990734));
#21630=CARTESIAN_POINT('Ctrl Pts',(-0.722004372559477,1.08536870078326,
2.16448346886966));
#21631=CARTESIAN_POINT('Ctrl Pts',(-0.596088708472957,1.14885423684131,
2.15663291783199));
#21632=CARTESIAN_POINT('Ctrl Pts',(-0.473680783866961,1.07884375413848,
2.14878236679431));
#21633=CARTESIAN_POINT('Ctrl Pts',(-0.464558934858572,0.938124319016692,
2.14093181575663));
#21634=CARTESIAN_POINT('Ctrl Pts',(-0.576903853974382,0.85289646424536,
2.13308126471895));
#21635=CARTESIAN_POINT('Ctrl Pts',(-0.709961944003222,0.899594560207548,
2.12523071368127));
#21636=CARTESIAN_POINT('Ctrl Pts',(-0.744403552230901,1.03633863630844,
2.1173801626436));
#21637=CARTESIAN_POINT('Ctrl Pts',(-0.64934061440031,1.14049336981984,2.10952961160591));
#21638=CARTESIAN_POINT('Ctrl Pts',(-0.510027855146882,1.11865028889668,
2.10167906056824));
#21639=CARTESIAN_POINT('Ctrl Pts',(-0.451404225723124,0.99039884810644,
2.09382850953056));
#21640=CARTESIAN_POINT('Ctrl Pts',(-0.526044875601709,0.87075787007063,
2.08597795849289));
#21641=CARTESIAN_POINT('Ctrl Pts',(-0.667010128672949,0.867024460974769,
2.0781274074552));
#21642=CARTESIAN_POINT('Ctrl Pts',(-0.747879322472409,0.982546373509308,
2.07027685641753));
#21643=CARTESIAN_POINT('Ctrl Pts',(-0.696126397524862,1.11372170867476,
2.06242630537985));
#21644=CARTESIAN_POINT('Ctrl Pts',(-0.558165872383014,1.14290754203214,
2.05457575434217));
#21645=CARTESIAN_POINT('Ctrl Pts',(-0.457721540280641,1.04393279273302,
2.04672520330449));
#21646=CARTESIAN_POINT('Ctrl Pts',(-0.484879149484439,0.905553554682652,
2.03887465226682));
#21647=CARTESIAN_POINT('Ctrl Pts',(-0.615273516218849,0.851885006312401,
2.03102410122914));
#21648=CARTESIAN_POINT('Ctrl Pts',(-0.731982722301914,0.931032073672457,
2.02317355019146));
#21649=CARTESIAN_POINT('Ctrl Pts',(-0.730302140552184,1.07206547359851,
2.01532299915378));
#21650=CARTESIAN_POINT('Ctrl Pts',(-0.611811749466523,1.14840144523713,
2.0074724481161));
#21651=CARTESIAN_POINT('Ctrl Pts',(-0.482633225963291,1.09178094916661,
1.99962189707843));
#21652=CARTESIAN_POINT('Ctrl Pts',(-0.45890197645103,0.952575083143895,
1.99177134604075));
#21653=CARTESIAN_POINT('Ctrl Pts',(-0.527170074345267,0.888579693265875,
1.98653764534896));
#21654=CARTESIAN_POINT('Ctrl Pts',(-0.56734149364689,0.877840168374445,
1.98392079500307));
#21655=CARTESIAN_POINT('Ctrl Pts',(-0.497154370004338,1.08857942294107,
2.40535973499898));
#21656=CARTESIAN_POINT('Ctrl Pts',(-0.468025636826573,1.05475934582637,
2.40274288465309));
#21657=CARTESIAN_POINT('Ctrl Pts',(-0.446190561956348,0.956718531983702,
2.3975091839613));
#21658=CARTESIAN_POINT('Ctrl Pts',(-0.551429149092544,0.847623301048373,
2.38965863292362));
#21659=CARTESIAN_POINT('Ctrl Pts',(-0.700229949071154,0.875541020369071,
2.38180808188594));
#21660=CARTESIAN_POINT('Ctrl Pts',(-0.759138563736414,1.01490064164717,
2.37395753084827));
#21661=CARTESIAN_POINT('Ctrl Pts',(-0.675329954255372,1.14098596339246,
2.36610697981059));
#21662=CARTESIAN_POINT('Ctrl Pts',(-0.523962603431266,1.14058649752482,
2.35825642877291));
#21663=CARTESIAN_POINT('Ctrl Pts',(-0.440787932286505,1.01412873225251,
2.35040587773523));
#21664=CARTESIAN_POINT('Ctrl Pts',(-0.500398156194616,0.874988270684254,
2.34255532669756));
#21665=CARTESIAN_POINT('Ctrl Pts',(-0.649333820146978,0.84796726183413,
2.33470477565988));
#21666=CARTESIAN_POINT('Ctrl Pts',(-0.754025670789615,0.957289792428312,
2.3268542246222));
#21667=CARTESIAN_POINT('Ctrl Pts',(-0.720583674030304,1.10491739707588,
2.31900367358452));
#21668=CARTESIAN_POINT('Ctrl Pts',(-0.578999353408684,1.15845179961484,
2.31115312254684));
#21669=CARTESIAN_POINT('Ctrl Pts',(-0.456248921215803,1.06988326141916,
2.30330257150917));
#21670=CARTESIAN_POINT('Ctrl Pts',(-0.462417869227328,0.918641549339655,
2.29545202047149));
#21671=CARTESIAN_POINT('Ctrl Pts',(-0.591973745354034,0.840364133660832,
2.28760146943381));
#21672=CARTESIAN_POINT('Ctrl Pts',(-0.728727756233707,0.905251905277888,
2.27975091839613));
#21673=CARTESIAN_POINT('Ctrl Pts',(-0.750035655620193,1.05511204760418,
2.27190036735845));
#21674=CARTESIAN_POINT('Ctrl Pts',(-0.636788011835149,1.15554638175604,
2.26404981632077));
#21675=CARTESIAN_POINT('Ctrl Pts',(-0.490548004613153,1.11648302980295,
2.2561992652831));
#21676=CARTESIAN_POINT('Ctrl Pts',(-0.442467148844067,0.972954923955743,
2.24834871424542));
#21677=CARTESIAN_POINT('Ctrl Pts',(-0.535665499162523,0.85368148706755,
2.24049816320774));
#21678=CARTESIAN_POINT('Ctrl Pts',(-0.686560559276222,0.865629970182854,
2.23264761217006));
#21679=CARTESIAN_POINT('Ctrl Pts',(-0.759826051981739,0.998084690970592,
2.22479706113239));
#21680=CARTESIAN_POINT('Ctrl Pts',(-0.689755741618848,1.13225710619039,
2.21694651009471));
#21681=CARTESIAN_POINT('Ctrl Pts',(-0.539190348351968,1.14781820447026,
2.20909595905703));
#21682=CARTESIAN_POINT('Ctrl Pts',(-0.443160496353055,1.03081242273638,
2.20124540801935));
#21683=CARTESIAN_POINT('Ctrl Pts',(-0.48778803986192,0.886173327813403,
2.19339485698167));
#21684=CARTESIAN_POINT('Ctrl Pts',(-0.633049936927148,0.843616698540163,
2.185544305944));
#21685=CARTESIAN_POINT('Ctrl Pts',(-0.748671864803154,0.941308331874462,
2.17769375490632));
#21686=CARTESIAN_POINT('Ctrl Pts',(-0.730961329922812,1.09163604839579,
2.16984320386864));
#21687=CARTESIAN_POINT('Ctrl Pts',(-0.595801560801866,1.15978237838877,
2.16199265283096));
#21688=CARTESIAN_POINT('Ctrl Pts',(-0.46440705203803,1.08463207245338,2.15414210179328));
#21689=CARTESIAN_POINT('Ctrl Pts',(-0.454615522009781,0.933581712675886,
2.14629155075561));
#21690=CARTESIAN_POINT('Ctrl Pts',(-0.575208249211462,0.842096850509319,
2.13844099971793));
#21691=CARTESIAN_POINT('Ctrl Pts',(-0.718034805847138,0.892223289617803,
2.13059044868025));
#21692=CARTESIAN_POINT('Ctrl Pts',(-0.755004946535977,1.03900643918491,
2.12273989764257));
#21693=CARTESIAN_POINT('Ctrl Pts',(-0.652962958175316,1.15080769787963,
2.11488934660489));
#21694=CARTESIAN_POINT('Ctrl Pts',(-0.503422545448295,1.12736100603329,
2.10703879556722));
#21695=CARTESIAN_POINT('Ctrl Pts',(-0.440495059218284,0.989693979040313,
2.09918824452954));
#21696=CARTESIAN_POINT('Ctrl Pts',(-0.520615456293703,0.861269552373166,
2.09133769349186));
#21697=CARTESIAN_POINT('Ctrl Pts',(-0.671929680758203,0.857262054854161,
2.08348714245418));
#21698=CARTESIAN_POINT('Ctrl Pts',(-0.758735890630724,0.98126501461181,
2.07563659141651));
#21699=CARTESIAN_POINT('Ctrl Pts',(-0.703183522003752,1.12207059383778,
2.06778604037882));
#21700=CARTESIAN_POINT('Ctrl Pts',(-0.555094617726015,1.15339910667059,
2.05993548934115));
#21701=CARTESIAN_POINT('Ctrl Pts',(-0.447276159752938,1.04715812099878,
2.05208493830347));
#21702=CARTESIAN_POINT('Ctrl Pts',(-0.476427546250332,0.89861976398254,
2.0442343872658));
#21703=CARTESIAN_POINT('Ctrl Pts',(-0.616394822207238,0.841011136339552,
2.03638383622811));
#21704=CARTESIAN_POINT('Ctrl Pts',(-0.74167224073109,0.925968789770463,
2.02853328519044));
#21705=CARTESIAN_POINT('Ctrl Pts',(-0.73986827898471,1.07735616409467,2.02068273415276));
#21706=CARTESIAN_POINT('Ctrl Pts',(-0.612678909668559,1.1592963450654,2.01283218311508));
#21707=CARTESIAN_POINT('Ctrl Pts',(-0.474016738136951,1.09851905232804,
2.0049816320774));
#21708=CARTESIAN_POINT('Ctrl Pts',(-0.448543257706232,0.949093380403833,
1.99713108103973));
#21709=CARTESIAN_POINT('Ctrl Pts',(-0.5218232615616,0.880399765646143,1.99189738034794));
#21710=CARTESIAN_POINT('Ctrl Pts',(-0.564943867702685,0.86887179797568,
1.98928053000205));
#21711=CARTESIAN_POINT('Ctrl Pts',(-0.490120355280912,1.09463771598849,
2.41071946999795));
#21712=CARTESIAN_POINT('Ctrl Pts',(-0.458999394158645,1.05850455157604,
2.40810261965206));
#21713=CARTESIAN_POINT('Ctrl Pts',(-0.435670933151054,0.953758343171685,
2.40286891896027));
#21714=CARTESIAN_POINT('Ctrl Pts',(-0.548107198705087,0.837201662871056,
2.3950183679226));
#21715=CARTESIAN_POINT('Ctrl Pts',(-0.707085067149817,0.867028784163962,
2.38716781688492));
#21716=CARTESIAN_POINT('Ctrl Pts',(-0.770022672282728,1.01591975478537,
2.37931726584724));
#21717=CARTESIAN_POINT('Ctrl Pts',(-0.680482064338898,1.15062854463137,
2.37146671480957));
#21718=CARTESIAN_POINT('Ctrl Pts',(-0.518762108602093,1.15020175773127,
2.36361616377188));
#21719=CARTESIAN_POINT('Ctrl Pts',(-0.429898796515824,1.01509505148933,
2.35576561273421));
#21720=CARTESIAN_POINT('Ctrl Pts',(-0.493585996690737,0.866438229767152,
2.34791506169653));
#21721=CARTESIAN_POINT('Ctrl Pts',(-0.652707952983651,0.837569148479711,
2.34006451065885));
#21722=CARTESIAN_POINT('Ctrl Pts',(-0.764560088597795,0.954368674351516,
2.33221395962117));
#21723=CARTESIAN_POINT('Ctrl Pts',(-0.728830862934391,1.11209310804976,
2.3243634085835));
#21724=CARTESIAN_POINT('Ctrl Pts',(-0.577563037083615,1.16928893767788,
2.31651285754582));
#21725=CARTESIAN_POINT('Ctrl Pts',(-0.446417222924693,1.07466285088508,
2.30866230650814));
#21726=CARTESIAN_POINT('Ctrl Pts',(-0.453008089409011,0.913077126817822,
2.30081175547046));
#21727=CARTESIAN_POINT('Ctrl Pts',(-0.591424798419137,0.829446012645248,
2.29296120443278));
#21728=CARTESIAN_POINT('Ctrl Pts',(-0.737531950760006,0.89877171265016,
2.28511065339511));
#21729=CARTESIAN_POINT('Ctrl Pts',(-0.760297180691466,1.05888137600737,
2.27726010235743));
#21730=CARTESIAN_POINT('Ctrl Pts',(-0.639304087791949,1.16618480693263,
2.26940955131975));
#21731=CARTESIAN_POINT('Ctrl Pts',(-0.483062154732201,1.12444975961634,
2.26155900028207));
#21732=CARTESIAN_POINT('Ctrl Pts',(-0.431692861258868,0.971105205468923,
2.25370844924439));
#21733=CARTESIAN_POINT('Ctrl Pts',(-0.531265411126364,0.843674191917333,
2.24585789820672));
#21734=CARTESIAN_POINT('Ctrl Pts',(-0.692480774344598,0.856439878506999,
2.23800734716904));
#21735=CARTESIAN_POINT('Ctrl Pts',(-0.770757180536974,0.997953695497927,
2.23015679613137));
#21736=CARTESIAN_POINT('Ctrl Pts',(-0.695894487699607,1.14130268675866,
2.22230624509368));
#21737=CARTESIAN_POINT('Ctrl Pts',(-0.53503133853272,1.15792806938798,2.21445569405601));
#21738=CARTESIAN_POINT('Ctrl Pts',(-0.432433629514727,1.03291980479239,
2.20660514301833));
#21739=CARTESIAN_POINT('Ctrl Pts',(-0.480113425201198,0.878388276682764,
2.19875459198065));
#21740=CARTESIAN_POINT('Ctrl Pts',(-0.635310351326514,0.83292103315299,
2.19090404094297));
#21741=CARTESIAN_POINT('Ctrl Pts',(-0.758840114888534,0.937294179228842,
2.18305348990529));
#21742=CARTESIAN_POINT('Ctrl Pts',(-0.739918287286149,1.09790339600832,
2.17520293886762));
#21743=CARTESIAN_POINT('Ctrl Pts',(-0.595514413130776,1.17071051993624,
2.16735238782994));
#21744=CARTESIAN_POINT('Ctrl Pts',(-0.455133320209099,1.09042039076827,
2.15950183679226));
#21745=CARTESIAN_POINT('Ctrl Pts',(-0.44467210916099,0.92903910633508,2.15165128575458));
#21746=CARTESIAN_POINT('Ctrl Pts',(-0.573512644448544,0.831297236773279,
2.14380073471691));
#21747=CARTESIAN_POINT('Ctrl Pts',(-0.726107667691055,0.884852019028058,
2.13595018367922));
#21748=CARTESIAN_POINT('Ctrl Pts',(-0.765606340841053,1.04167424206138,
2.12809963264155));
#21749=CARTESIAN_POINT('Ctrl Pts',(-0.656585301950322,1.16112202593943,
2.12024908160387));
#21750=CARTESIAN_POINT('Ctrl Pts',(-0.496817235749707,1.1360717231699,2.11239853056619));
#21751=CARTESIAN_POINT('Ctrl Pts',(-0.429585892713444,0.988989109974185,
2.10454797952851));
#21752=CARTESIAN_POINT('Ctrl Pts',(-0.515186036985696,0.851781234675702,
2.09669742849084));
#21753=CARTESIAN_POINT('Ctrl Pts',(-0.67684923284346,0.847499648733552,
2.08884687745316));
#21754=CARTESIAN_POINT('Ctrl Pts',(-0.769592458789038,0.979983655714312,
2.08099632641548));
#21755=CARTESIAN_POINT('Ctrl Pts',(-0.710240646482644,1.1304194790008,2.0731457753778));
#21756=CARTESIAN_POINT('Ctrl Pts',(-0.552023363069014,1.16389067130903,
2.06529522434013));
#21757=CARTESIAN_POINT('Ctrl Pts',(-0.436830779225235,1.05038344926453,
2.05744467330245));
#21758=CARTESIAN_POINT('Ctrl Pts',(-0.467975943016225,0.891685973282426,
2.04959412226477));
#21759=CARTESIAN_POINT('Ctrl Pts',(-0.617516128195625,0.830137266366705,
2.04174357122709));
#21760=CARTESIAN_POINT('Ctrl Pts',(-0.751361759160267,0.920905505868468,
2.03389302018941));
#21761=CARTESIAN_POINT('Ctrl Pts',(-0.749434417417234,1.08264685459083,
2.02604246915173));
#21762=CARTESIAN_POINT('Ctrl Pts',(-0.613546069870597,1.17019124489367,
2.01819191811406));
#21763=CARTESIAN_POINT('Ctrl Pts',(-0.465400250310609,1.10525715548948,
2.01034136707638));
#21764=CARTESIAN_POINT('Ctrl Pts',(-0.438184538961436,0.945611677663771,
2.0024908160387));
#21765=CARTESIAN_POINT('Ctrl Pts',(-0.516476448777932,0.872219838026411,
1.99725711534692));
#21766=CARTESIAN_POINT('Ctrl Pts',(-0.56254624175848,0.859903427576914,
1.99464026500102));
#21767=CARTESIAN_POINT('Ctrl Pts',(-0.483086340557485,1.10069600903591,
2.41607920499693));
#21768=CARTESIAN_POINT('Ctrl Pts',(-0.449973151490718,1.0622497573257,2.41346235465104));
#21769=CARTESIAN_POINT('Ctrl Pts',(-0.42515130434576,0.950798154359666,
2.40822865395925));
#21770=CARTESIAN_POINT('Ctrl Pts',(-0.54478524831763,0.826780024693742,
2.40037810292158));
#21771=CARTESIAN_POINT('Ctrl Pts',(-0.71394018522848,0.858516547958849,
2.3925275518839));
#21772=CARTESIAN_POINT('Ctrl Pts',(-0.780906780829043,1.01693886792356,
2.38467700084622));
#21773=CARTESIAN_POINT('Ctrl Pts',(-0.685634174422424,1.16027112587027,
2.37682644980854));
#21774=CARTESIAN_POINT('Ctrl Pts',(-0.513561613772921,1.15981701793772,
2.36897589877087));
#21775=CARTESIAN_POINT('Ctrl Pts',(-0.419009660745144,1.01606137072615,
2.36112534773318));
#21776=CARTESIAN_POINT('Ctrl Pts',(-0.486773837186857,0.857888188850051,
2.35327479669551));
#21777=CARTESIAN_POINT('Ctrl Pts',(-0.656082085820325,0.827171035125292,
2.34542424565783));
#21778=CARTESIAN_POINT('Ctrl Pts',(-0.775094506405975,0.951447556274721,
2.33757369462015));
#21779=CARTESIAN_POINT('Ctrl Pts',(-0.737078051838477,1.11926881902364,
2.32972314358247));
#21780=CARTESIAN_POINT('Ctrl Pts',(-0.576126720758545,1.18012607574093,
2.3218725925448));
#21781=CARTESIAN_POINT('Ctrl Pts',(-0.436585524633584,1.079442440351,2.31402204150712));
#21782=CARTESIAN_POINT('Ctrl Pts',(-0.443598309590693,0.907512704295987,
2.30617149046944));
#21783=CARTESIAN_POINT('Ctrl Pts',(-0.59087585148424,0.818527891629664,
2.29832093943176));
#21784=CARTESIAN_POINT('Ctrl Pts',(-0.746336145286304,0.892291520022432,
2.29047038839408));
#21785=CARTESIAN_POINT('Ctrl Pts',(-0.77055870576274,1.06265070441055,2.28261983735641));
#21786=CARTESIAN_POINT('Ctrl Pts',(-0.641820163748749,1.17682323210921,
2.27476928631873));
#21787=CARTESIAN_POINT('Ctrl Pts',(-0.47557630485125,1.13241648942973,2.26691873528105));
#21788=CARTESIAN_POINT('Ctrl Pts',(-0.420918573673669,0.969255486982105,
2.25906818424337));
#21789=CARTESIAN_POINT('Ctrl Pts',(-0.526865323090207,0.833666896767115,
2.2512176332057));
#21790=CARTESIAN_POINT('Ctrl Pts',(-0.698400989412974,0.847249786831145,
2.24336708216802));
#21791=CARTESIAN_POINT('Ctrl Pts',(-0.781688309092209,0.997822700025263,
2.23551653113034));
#21792=CARTESIAN_POINT('Ctrl Pts',(-0.702033233780365,1.15034826732694,
2.22766598009266));
#21793=CARTESIAN_POINT('Ctrl Pts',(-0.530872328713473,1.16803793430571,
2.21981542905499));
#21794=CARTESIAN_POINT('Ctrl Pts',(-0.421706762676398,1.0350271868484,2.2119648780173));
#21795=CARTESIAN_POINT('Ctrl Pts',(-0.472438810540477,0.870603225552124,
2.20411432697963));
#21796=CARTESIAN_POINT('Ctrl Pts',(-0.637570765725878,0.822225367765818,
2.19626377594195));
#21797=CARTESIAN_POINT('Ctrl Pts',(-0.769008364973917,0.933280026583224,
2.18841322490427));
#21798=CARTESIAN_POINT('Ctrl Pts',(-0.748875244649484,1.10417074362085,
2.18056267386659));
#21799=CARTESIAN_POINT('Ctrl Pts',(-0.595227265459685,1.1816386614837,2.17271212282892));
#21800=CARTESIAN_POINT('Ctrl Pts',(-0.445859588380167,1.09620870908317,
2.16486157179124));
#21801=CARTESIAN_POINT('Ctrl Pts',(-0.434728696312199,0.924496499994273,
2.15701102075356));
#21802=CARTESIAN_POINT('Ctrl Pts',(-0.571817039685625,0.820497623037239,
2.14916046971588));
#21803=CARTESIAN_POINT('Ctrl Pts',(-0.734180529534971,0.877480748438312,
2.14130991867821));
#21804=CARTESIAN_POINT('Ctrl Pts',(-0.776207735146129,1.04434204493786,
2.13345936764052));
#21805=CARTESIAN_POINT('Ctrl Pts',(-0.660207645725328,1.17143635399922,
2.12560881660285));
#21806=CARTESIAN_POINT('Ctrl Pts',(-0.490211926051119,1.14478244030651,
2.11775826556517));
#21807=CARTESIAN_POINT('Ctrl Pts',(-0.418676726208604,0.988284240908056,
2.10990771452749));
#21808=CARTESIAN_POINT('Ctrl Pts',(-0.509756617677689,0.842292916978238,
2.10205716348981));
#21809=CARTESIAN_POINT('Ctrl Pts',(-0.681768784928714,0.837737242612945,
2.09420661245213));
#21810=CARTESIAN_POINT('Ctrl Pts',(-0.780449026947353,0.978702296816814,
2.08635606141446));
#21811=CARTESIAN_POINT('Ctrl Pts',(-0.717297770961535,1.13876836416382,
2.07850551037678));
#21812=CARTESIAN_POINT('Ctrl Pts',(-0.548952108412014,1.17438223594748,
2.0706549593391));
#21813=CARTESIAN_POINT('Ctrl Pts',(-0.426385398697532,1.05360877753029,
2.06280440830142));
#21814=CARTESIAN_POINT('Ctrl Pts',(-0.459524339782119,0.884752182582313,
2.05495385726375));
#21815=CARTESIAN_POINT('Ctrl Pts',(-0.618637434184013,0.819263396393857,
2.04710330622607));
#21816=CARTESIAN_POINT('Ctrl Pts',(-0.761051277589445,0.915842221966472,
2.03925275518839));
#21817=CARTESIAN_POINT('Ctrl Pts',(-0.759000555849758,1.08793754508699,
2.03140220415071));
#21818=CARTESIAN_POINT('Ctrl Pts',(-0.614413230072635,1.18108614472194,
2.02355165311304));
#21819=CARTESIAN_POINT('Ctrl Pts',(-0.456783762484268,1.11199525865091,
2.01570110207535));
#21820=CARTESIAN_POINT('Ctrl Pts',(-0.427825820216639,0.942129974923708,
2.00785055103768));
#21821=CARTESIAN_POINT('Ctrl Pts',(-0.511129635994264,0.864039910406679,
2.00261685034589));
#21822=CARTESIAN_POINT('Ctrl Pts',(-0.560148615814275,0.850935057178149,
2.));
#21823=CARTESIAN_POINT('Ctrl Pts',(-0.560148615814275,0.850935057178149,
2.));
#21824=CARTESIAN_POINT('Ctrl Pts',(-0.550119441743087,0.85459967610481,
2.));
#21825=CARTESIAN_POINT('Ctrl Pts',(-0.540564999899567,0.859362631836586,
2.));
#21826=CARTESIAN_POINT('Ctrl Pts',(-0.531596825272739,0.86507409197529,
2.));
#21827=CARTESIAN_POINT('Ctrl Pts',(-0.527131635014649,0.867917787290334,
2.));
#21828=CARTESIAN_POINT('Ctrl Pts',(-0.522812202969371,0.870997335784893,
2.));
#21829=CARTESIAN_POINT('Ctrl Pts',(-0.518655551555349,0.874297548143145,
2.));
#21830=CARTESIAN_POINT('Ctrl Pts',(-0.515850210886717,0.876524874666724,
2.));
#21831=CARTESIAN_POINT('Ctrl Pts',(-0.51311906464033,0.878852752659134,
2.));
#21832=CARTESIAN_POINT('Ctrl Pts',(-0.510468070497139,0.881276854651557,
2.));
#21833=CARTESIAN_POINT('Ctrl Pts',(-0.508096882944962,0.883445098019579,
2.));
#21834=CARTESIAN_POINT('Ctrl Pts',(-0.505796523707934,0.885684247113283,
2.));
#21835=CARTESIAN_POINT('Ctrl Pts',(-0.503571407093493,0.887989067169883,
2.));
#21836=CARTESIAN_POINT('Ctrl Pts',(-0.496344337828248,0.895475009293033,
2.));
#21837=CARTESIAN_POINT('Ctrl Pts',(-0.489902887206981,0.90365635994166,
2.));
#21838=CARTESIAN_POINT('Ctrl Pts',(-0.4843803033401,0.912413093858066,2.));
#21839=CARTESIAN_POINT('Ctrl Pts',(-0.482085852075076,0.91605122769112,
2.));
#21840=CARTESIAN_POINT('Ctrl Pts',(-0.479950567463666,0.919788922535331,
2.));
#21841=CARTESIAN_POINT('Ctrl Pts',(-0.477986666560954,0.923618208076587,
2.));
#21842=CARTESIAN_POINT('Ctrl Pts',(-0.47650289740366,0.926511315245457,
2.));
#21843=CARTESIAN_POINT('Ctrl Pts',(-0.475117210175375,0.929457020402162,
2.));
#21844=CARTESIAN_POINT('Ctrl Pts',(-0.473840374763333,0.932438174193855,
2.));
#21845=CARTESIAN_POINT('Ctrl Pts',(-0.470678071962382,0.939821514988315,
2.));
#21846=CARTESIAN_POINT('Ctrl Pts',(-0.468171074744705,0.947441922900028,
2.));
#21847=CARTESIAN_POINT('Ctrl Pts',(-0.466390213028648,0.95524361805541,
2.));
#21848=CARTESIAN_POINT('Ctrl Pts',(-0.464752059680358,0.962420128688376,
2.));
#21849=CARTESIAN_POINT('Ctrl Pts',(-0.463728780577517,0.969750541677906,
2.));
#21850=CARTESIAN_POINT('Ctrl Pts',(-0.463308983993722,0.977159407672611,
2.));
#21851=CARTESIAN_POINT('Ctrl Pts',(-0.46313283978449,0.9802681248283,2.));
#21852=CARTESIAN_POINT('Ctrl Pts',(-0.463063521137214,0.983387155046876,
2.));
#21853=CARTESIAN_POINT('Ctrl Pts',(-0.463099420187341,0.986501027428933,
2.));
#21854=CARTESIAN_POINT('Ctrl Pts',(-0.463196744049792,0.994942868824082,
2.));
#21855=CARTESIAN_POINT('Ctrl Pts',(-0.464064111260558,1.00336874731576,
2.));
#21856=CARTESIAN_POINT('Ctrl Pts',(-0.465675457037548,1.01166504030789,
2.));
#21857=CARTESIAN_POINT('Ctrl Pts',(-0.466871286975471,1.01782197799031,
2.));
#21858=CARTESIAN_POINT('Ctrl Pts',(-0.468477483228933,1.02390757245997,
2.));
#21859=CARTESIAN_POINT('Ctrl Pts',(-0.47049180892072,1.02987016754483,2.));
#21860=CARTESIAN_POINT('Ctrl Pts',(-0.471677004317114,1.03337845832122,
2.));
#21861=CARTESIAN_POINT('Ctrl Pts',(-0.473001297362186,1.03683670978256,
2.));
#21862=CARTESIAN_POINT('Ctrl Pts',(-0.474460925722079,1.04022912201569,
2.));
#21863=CARTESIAN_POINT('Ctrl Pts',(-0.476751357662528,1.04555245605566,
2.));
#21864=CARTESIAN_POINT('Ctrl Pts',(-0.479376312983413,1.05071850549913,
2.));
#21865=CARTESIAN_POINT('Ctrl Pts',(-0.482333055615295,1.05568494193306,
2.));
#21866=CARTESIAN_POINT('Ctrl Pts',(-0.484374509820886,1.05911396968661,
2.));
#21867=CARTESIAN_POINT('Ctrl Pts',(-0.486574680171624,1.06244757845398,
2.));
#21868=CARTESIAN_POINT('Ctrl Pts',(-0.488924280031899,1.0656592034053,2.));
#21869=CARTESIAN_POINT('Ctrl Pts',(-0.492216707647991,1.07015956232216,
2.));
#21870=CARTESIAN_POINT('Ctrl Pts',(-0.495805970213506,1.07442716727356,
2.));
#21871=CARTESIAN_POINT('Ctrl Pts',(-0.499690940637682,1.07842077494232,
2.));
#21872=CARTESIAN_POINT('Ctrl Pts',(-0.501092717011139,1.07986174984398,
2.));
#21873=CARTESIAN_POINT('Ctrl Pts',(-0.502533033199793,1.08126699098065,
2.));
#21874=CARTESIAN_POINT('Ctrl Pts',(-0.504010174669742,1.08263575197434,
2.));
#21875=CARTESIAN_POINT('Ctrl Pts',(-0.504188384727764,1.08252112989365,
2.4));
#21876=CARTESIAN_POINT('Ctrl Pts',(-0.497506954663502,1.07628156217526,
2.4));
#21877=CARTESIAN_POINT('Ctrl Pts',(-0.491604269963233,1.06931033894935,
2.4));
#21878=CARTESIAN_POINT('Ctrl Pts',(-0.48648731081533,1.06178682142811,2.4));
#21879=CARTESIAN_POINT('Ctrl Pts',(-0.482497621478512,1.05592074027282,
2.4));
#21880=CARTESIAN_POINT('Ctrl Pts',(-0.478985885254584,1.04971755224006,
2.4));
#21881=CARTESIAN_POINT('Ctrl Pts',(-0.475968008505373,1.04324617240972,
2.4));
#21882=CARTESIAN_POINT('Ctrl Pts',(-0.474670784833122,1.04046447262352,
2.4));
#21883=CARTESIAN_POINT('Ctrl Pts',(-0.473467326409776,1.03763771123602,
2.4));
#21884=CARTESIAN_POINT('Ctrl Pts',(-0.472361166010358,1.03477908326479,
2.4));
#21885=CARTESIAN_POINT('Ctrl Pts',(-0.46880698586937,1.02559408733548,2.4));
#21886=CARTESIAN_POINT('Ctrl Pts',(-0.466243719906724,1.01606060675579,
2.4));
#21887=CARTESIAN_POINT('Ctrl Pts',(-0.464705314070165,1.00636042835626,
2.4));
#21888=CARTESIAN_POINT('Ctrl Pts',(-0.463992227392452,1.00186417137142,
2.4));
#21889=CARTESIAN_POINT('Ctrl Pts',(-0.463499928942431,0.997331640290426,
2.4));
#21890=CARTESIAN_POINT('Ctrl Pts',(-0.463235268916811,0.992779403524773,
2.4));
#21891=CARTESIAN_POINT('Ctrl Pts',(-0.463040851274643,0.989435358134849,
2.4));
#21892=CARTESIAN_POINT('Ctrl Pts',(-0.462969940004504,0.986088143884579,
2.4));
#21893=CARTESIAN_POINT('Ctrl Pts',(-0.463023793901296,0.982751466845985,
2.4));
#21894=CARTESIAN_POINT('Ctrl Pts',(-0.463137062422501,0.975733581485534,
2.4));
#21895=CARTESIAN_POINT('Ctrl Pts',(-0.463800894161501,0.968753185610107,
2.4));
#21896=CARTESIAN_POINT('Ctrl Pts',(-0.465031332332612,0.96187163776825,
2.4));
#21897=CARTESIAN_POINT('Ctrl Pts',(-0.466389645164331,0.954274917384296,
2.4));
#21898=CARTESIAN_POINT('Ctrl Pts',(-0.468438000905081,0.946798204321114,
2.4));
#21899=CARTESIAN_POINT('Ctrl Pts',(-0.471116528460654,0.93949859713407,
2.4));
#21900=CARTESIAN_POINT('Ctrl Pts',(-0.472251134057494,0.936406534425243,
2.4));
#21901=CARTESIAN_POINT('Ctrl Pts',(-0.473496260389133,0.933354194164882,
2.4));
#21902=CARTESIAN_POINT('Ctrl Pts',(-0.474844488633202,0.930349739998837,
2.4));
#21903=CARTESIAN_POINT('Ctrl Pts',(-0.478666411965482,0.9218327893056,2.4));
#21904=CARTESIAN_POINT('Ctrl Pts',(-0.4833179823867,0.913689872025069,2.4));
#21905=CARTESIAN_POINT('Ctrl Pts',(-0.488689869589499,0.906016299690457,
2.4));
#21906=CARTESIAN_POINT('Ctrl Pts',(-0.491565626713204,0.901908370861642,
2.4));
#21907=CARTESIAN_POINT('Ctrl Pts',(-0.494648453197326,0.897935009702848,
2.4));
#21908=CARTESIAN_POINT('Ctrl Pts',(-0.497925430586844,0.894112166139119,
2.4));
#21909=CARTESIAN_POINT('Ctrl Pts',(-0.500336511660046,0.89129945653917,
2.4));
#21910=CARTESIAN_POINT('Ctrl Pts',(-0.502853434868661,0.888568042774596,
2.4));
#21911=CARTESIAN_POINT('Ctrl Pts',(-0.505459753140441,0.885935602377086,
2.4));
#21912=CARTESIAN_POINT('Ctrl Pts',(-0.510032980818731,0.881316538996496,
2.4));
#21913=CARTESIAN_POINT('Ctrl Pts',(-0.514888373574847,0.876993017632294,
2.4));
#21914=CARTESIAN_POINT('Ctrl Pts',(-0.519995790255463,0.872997627556259,
2.4));
#21915=CARTESIAN_POINT('Ctrl Pts',(-0.524771384850184,0.869261812672909,
2.4));
#21916=CARTESIAN_POINT('Ctrl Pts',(-0.529772960099733,0.865810225418053,
2.4));
#21917=CARTESIAN_POINT('Ctrl Pts',(-0.534950219195867,0.86268896384257,
2.4));
#21918=CARTESIAN_POINT('Ctrl Pts',(-0.540826101062414,0.859146517163432,
2.4));
#21919=CARTESIAN_POINT('Ctrl Pts',(-0.546932707573367,0.85602468566073,
2.4));
#21920=CARTESIAN_POINT('Ctrl Pts',(-0.553238064171717,0.853364150883981,
2.4));
#21921=CARTESIAN_POINT('Ctrl Pts',(-0.555483414843566,0.852416728885673,
2.4));
#21922=CARTESIAN_POINT('Ctrl Pts',(-0.557754020887936,0.851527863380312,
2.4));
#21923=CARTESIAN_POINT('Ctrl Pts',(-0.560047768817924,0.850696978396871,
2.4));
#21924=CARTESIAN_POINT('Ctrl Pts',(-0.72640212307541,0.999893075304641,
2.31934196736194));
#21925=CARTESIAN_POINT('Ctrl Pts',(-0.726497678848041,0.988483569383442,
2.32005947478237));
#21926=CARTESIAN_POINT('Ctrl Pts',(-0.725076811113891,0.977097445695636,
2.32077698220279));
#21927=CARTESIAN_POINT('Ctrl Pts',(-0.722043530727044,0.966158450551832,
2.32149448962322));
#21928=CARTESIAN_POINT('Ctrl Pts',(-0.710980731091059,0.926262398732923,
2.32411133996911));
#21929=CARTESIAN_POINT('Ctrl Pts',(-0.678470209200682,0.892313886960735,
2.32672819031501));
#21930=CARTESIAN_POINT('Ctrl Pts',(-0.639090052986859,0.879535120476776,
2.3293450406609));
#21931=CARTESIAN_POINT('Ctrl Pts',(-0.599709896773035,0.866756353992817,
2.33196189100679));
#21932=CARTESIAN_POINT('Ctrl Pts',(-0.553460106235766,0.875147332797086,
2.33457874135268));
#21933=CARTESIAN_POINT('Ctrl Pts',(-0.52107966969358,0.900946839101611,
2.33719559169858));
#21934=CARTESIAN_POINT('Ctrl Pts',(-0.488699233151393,0.926746345406136,
2.33981244204447));
#21935=CARTESIAN_POINT('Ctrl Pts',(-0.470188150604288,0.969954379210915,
2.34242929239036));
#21936=CARTESIAN_POINT('Ctrl Pts',(-0.473846947697945,1.01119320016375,
2.34504614273626));
#21937=CARTESIAN_POINT('Ctrl Pts',(-0.477505744791602,1.05243202111659,
2.34766299308215));
#21938=CARTESIAN_POINT('Ctrl Pts',(-0.503334421526021,1.09170162921748,
2.35027984342804));
#21939=CARTESIAN_POINT('Ctrl Pts',(-0.539751217545131,1.11139845740712,
2.35289669377393));
#21940=CARTESIAN_POINT('Ctrl Pts',(-0.576168013564241,1.13109528559677,
2.35551354411982));
#21941=CARTESIAN_POINT('Ctrl Pts',(-0.623172928868043,1.13121933387517,
2.35813039446572));
#21942=CARTESIAN_POINT('Ctrl Pts',(-0.659688155022986,1.11170438240693,
2.36074724481161));
#21943=CARTESIAN_POINT('Ctrl Pts',(-0.696203381177929,1.0921894309387,2.3633640951575));
#21944=CARTESIAN_POINT('Ctrl Pts',(-0.722228918184014,1.05303547972384,
2.3659809455034));
#21945=CARTESIAN_POINT('Ctrl Pts',(-0.726095082654122,1.01182045879394,
2.36859779584929));
#21946=CARTESIAN_POINT('Ctrl Pts',(-0.726461565140266,1.00791359361693,
2.36884585302017));
#21947=CARTESIAN_POINT('Ctrl Pts',(-0.726628932956602,1.00398820854659,
2.36909391019106));
#21948=CARTESIAN_POINT('Ctrl Pts',(-0.726604172280256,1.00006079745576,
2.36934196736194));
#21949=CARTESIAN_POINT('Ctrl Pts',(-0.639851384185722,0.850935057178148,
2.4));
#21950=CARTESIAN_POINT('Ctrl Pts',(-0.688870364005733,0.864039910406677,
2.39738314965411));
#21951=CARTESIAN_POINT('Ctrl Pts',(-0.772174172732383,0.942130018479807,
2.39214944896232));
#21952=CARTESIAN_POINT('Ctrl Pts',(-0.743216243669936,1.11199523763249,
2.38429889792464));
#21953=CARTESIAN_POINT('Ctrl Pts',(-0.585586769094172,1.18108616109394,
2.37644834688697));
#21954=CARTESIAN_POINT('Ctrl Pts',(-0.44099944093888,1.08793753892263,2.36859779584929));
#21955=CARTESIAN_POINT('Ctrl Pts',(-0.438948720197302,0.915842224941729,
2.36074724481161));
#21956=CARTESIAN_POINT('Ctrl Pts',(-0.581362564989717,0.819263390701727,
2.35289669377393));
#21957=CARTESIAN_POINT('Ctrl Pts',(-0.740475663026546,0.88475218199663,
2.34504614273626));
#21958=CARTESIAN_POINT('Ctrl Pts',(-0.773614604105453,1.05360877766967,
2.33719559169858));
#21959=CARTESIAN_POINT('Ctrl Pts',(-0.651047892623131,1.17438223943631,
2.3293450406609));
#21960=CARTESIAN_POINT('Ctrl Pts',(-0.48270222690289,1.13876836634555,2.32149448962322));
#21961=CARTESIAN_POINT('Ctrl Pts',(-0.419550969949932,0.978702296577685,
2.31364393858554));
#21962=CARTESIAN_POINT('Ctrl Pts',(-0.518231213613428,0.837737239705173,
2.30579338754787));
#21963=CARTESIAN_POINT('Ctrl Pts',(-0.690243383915708,0.842292914261777,
2.29794283651019));
#21964=CARTESIAN_POINT('Ctrl Pts',(-0.781323276950512,0.988284240682119,
2.29009228547251));
#21965=CARTESIAN_POINT('Ctrl Pts',(-0.709788075872465,1.14478244284782,
2.28224173443483));
#21966=CARTESIAN_POINT('Ctrl Pts',(-0.539792353219763,1.17143635698873,
2.27439118339715));
#21967=CARTESIAN_POINT('Ctrl Pts',(-0.423792261776434,1.04434204571596,
2.26654063235948));
#21968=CARTESIAN_POINT('Ctrl Pts',(-0.465819468119529,0.877480746295693,
2.2586900813218));
#21969=CARTESIAN_POINT('Ctrl Pts',(-0.6281829608073,0.820497619901593,2.25083953028412));
#21970=CARTESIAN_POINT('Ctrl Pts',(-0.765271306575456,0.924496498674441,
2.24298897924644));
#21971=CARTESIAN_POINT('Ctrl Pts',(-0.754140414313383,1.09620871076456,
2.23513842820876));
#21972=CARTESIAN_POINT('Ctrl Pts',(-0.604772734623643,1.18163866465747,
2.22728787717109));
#21973=CARTESIAN_POINT('Ctrl Pts',(-0.451124752749149,1.10417074544119,
2.21943732613341));
#21974=CARTESIAN_POINT('Ctrl Pts',(-0.43099163207285,0.933280025417337,
2.21158677509573));
#21975=CARTESIAN_POINT('Ctrl Pts',(-0.562429233617627,0.822225364659454,
2.20373622405805));
#21976=CARTESIAN_POINT('Ctrl Pts',(-0.727561191688486,0.870603223291056,
2.19588567302038));
#21977=CARTESIAN_POINT('Ctrl Pts',(-0.778293240439059,1.03502718746047,
2.1880351219827));
#21978=CARTESIAN_POINT('Ctrl Pts',(-0.669127672494447,1.16803793724193,
2.18018457094502));
#21979=CARTESIAN_POINT('Ctrl Pts',(-0.497966764436741,1.15034826995414,
2.17233401990734));
#21980=CARTESIAN_POINT('Ctrl Pts',(-0.418311687733005,0.997822699987136,
2.16448346886966));
#21981=CARTESIAN_POINT('Ctrl Pts',(-0.501599008867606,0.847249784162188,
2.15663291783199));
#21982=CARTESIAN_POINT('Ctrl Pts',(-0.673134678187691,0.833666893860354,
2.1487823667943));
#21983=CARTESIAN_POINT('Ctrl Pts',(-0.779081429455625,0.969255486445431,
2.14093181575663));
#21984=CARTESIAN_POINT('Ctrl Pts',(-0.724423697322763,1.1324164917425,2.13308126471895));
#21985=CARTESIAN_POINT('Ctrl Pts',(-0.558179835520779,1.17682323520091,
2.12523071368127));
#21986=CARTESIAN_POINT('Ctrl Pts',(-0.429441291256411,1.0626507055017,2.1173801626436));
#21987=CARTESIAN_POINT('Ctrl Pts',(-0.453663852157743,0.892291518147041,
2.10952961160592));
#21988=CARTESIAN_POINT('Ctrl Pts',(-0.609124148673025,0.818527888446316,
2.10167906056824));
#21989=CARTESIAN_POINT('Ctrl Pts',(-0.756401693146515,0.907512702702641,
2.09382850953056));
#21990=CARTESIAN_POINT('Ctrl Pts',(-0.763414478213392,1.07944244169741,
2.08597795849288));
#21991=CARTESIAN_POINT('Ctrl Pts',(-0.623873279675432,1.18012607896462,
2.0781274074552));
#21992=CARTESIAN_POINT('Ctrl Pts',(-0.462921945732953,1.11926882096942,
2.07027685641753));
#21993=CARTESIAN_POINT('Ctrl Pts',(-0.424905490600427,0.951447555675582,
2.06242630537985));
#21994=CARTESIAN_POINT('Ctrl Pts',(-0.54391791306908,0.827171031659744,
2.05457575434217));
#21995=CARTESIAN_POINT('Ctrl Pts',(-0.713226165050295,0.857888187155562,
2.04672520330449));
#21996=CARTESIAN_POINT('Ctrl Pts',(-0.780990341905239,1.01606136962747,
2.03887465226682));
#21997=CARTESIAN_POINT('Ctrl Pts',(-0.686438388751686,1.15981702310584,
2.03102410122914));
#21998=CARTESIAN_POINT('Ctrl Pts',(-0.514365822072695,1.16027112465931,
2.02317355019146));
#21999=CARTESIAN_POINT('Ctrl Pts',(-0.41909321999119,1.01693887482571,2.01532299915378));
#22000=CARTESIAN_POINT('Ctrl Pts',(-0.486059804858393,0.858516534902566,
2.0074724481161));
#22001=CARTESIAN_POINT('Ctrl Pts',(-0.655214768609463,0.826780038590561,
1.99962189707843));
#22002=CARTESIAN_POINT('Ctrl Pts',(-0.774848665287453,0.950798122348591,
1.99177134604075));
#22003=CARTESIAN_POINT('Ctrl Pts',(-0.750026848509283,1.0622497573257,1.98653764534896));
#22004=CARTESIAN_POINT('Ctrl Pts',(-0.716913659442517,1.10069600903591,
1.98392079500307));
#22005=CARTESIAN_POINT('Ctrl Pts',(-0.637453758241517,0.859903427576914,
2.40535973499898));
#22006=CARTESIAN_POINT('Ctrl Pts',(-0.683523551222066,0.872219838026409,
2.40274288465309));
#22007=CARTESIAN_POINT('Ctrl Pts',(-0.761815454411802,0.945611718599352,
2.3975091839613));
#22008=CARTESIAN_POINT('Ctrl Pts',(-0.734599755473333,1.10525713573561,
2.38965863292362));
#22009=CARTESIAN_POINT('Ctrl Pts',(-0.586453929346337,1.17019126028066,
2.38180808188594));
#22010=CARTESIAN_POINT('Ctrl Pts',(-0.450565579564614,1.08264684879734,
2.37395753084827));
#22011=CARTESIAN_POINT('Ctrl Pts',(-0.448638238759637,0.920905508664721,
2.36610697981058));
#22012=CARTESIAN_POINT('Ctrl Pts',(-0.582483871027817,0.830137261017037,
2.35825642877291));
#22013=CARTESIAN_POINT('Ctrl Pts',(-0.732024059623459,0.891685972731981,
2.35040587773523));
#22014=CARTESIAN_POINT('Ctrl Pts',(-0.76316922340911,1.05038344939552,2.34255532669756));
#22015=CARTESIAN_POINT('Ctrl Pts',(-0.647976637903853,1.16389067458796,
2.33470477565988));
#22016=CARTESIAN_POINT('Ctrl Pts',(-0.489759351510266,1.13041948105126,
2.3268542246222));
#22017=CARTESIAN_POINT('Ctrl Pts',(-0.430407538294919,0.979983655489569,
2.31900367358452));
#22018=CARTESIAN_POINT('Ctrl Pts',(-0.523150765786394,0.847499646000726,
2.31115312254684));
#22019=CARTESIAN_POINT('Ctrl Pts',(-0.684813964511835,0.851781232122674,
2.30330257150917));
#22020=CARTESIAN_POINT('Ctrl Pts',(-0.770414110255606,0.98898910976184,
2.29545202047149));
#22021=CARTESIAN_POINT('Ctrl Pts',(-0.703182766058146,1.13607172555832,
2.28760146943381));
#22022=CARTESIAN_POINT('Ctrl Pts',(-0.543414697058237,1.16112202874907,
2.27975091839613));
#22023=CARTESIAN_POINT('Ctrl Pts',(-0.434393656266662,1.04167424279268,
2.27190036735845));
#22024=CARTESIAN_POINT('Ctrl Pts',(-0.47389233010456,0.884852017014347,
2.26404981632077));
#22025=CARTESIAN_POINT('Ctrl Pts',(-0.626487356014725,0.831297233826287,
2.2561992652831));
#22026=CARTESIAN_POINT('Ctrl Pts',(-0.755327893552931,0.929039105094654,
2.24834871424542));
#22027=CARTESIAN_POINT('Ctrl Pts',(-0.744866682322397,1.0904203923485,2.24049816320774));
#22028=CARTESIAN_POINT('Ctrl Pts',(-0.604485586947538,1.17071052291906,
2.23264761217006));
#22029=CARTESIAN_POINT('Ctrl Pts',(-0.460081710268994,1.09790339771914,
2.22479706113239));
#22030=CARTESIAN_POINT('Ctrl Pts',(-0.441159882335912,0.937294178133102,
2.21694651009471));
#22031=CARTESIAN_POINT('Ctrl Pts',(-0.564689648056489,0.832921030233517,
2.20909595905703));
#22032=CARTESIAN_POINT('Ctrl Pts',(-0.719886576893662,0.878388274557731,
2.20124540801935));
#22033=CARTESIAN_POINT('Ctrl Pts',(-0.767566373413291,1.03291980536764,
2.19339485698167));
#22034=CARTESIAN_POINT('Ctrl Pts',(-0.664968662602526,1.15792807214755,
2.185544305944));
#22035=CARTESIAN_POINT('Ctrl Pts',(-0.504105510624766,1.1413026892278,2.17769375490632));
#22036=CARTESIAN_POINT('Ctrl Pts',(-0.429242816479248,0.997953695462094,
2.16984320386864));
#22037=CARTESIAN_POINT('Ctrl Pts',(-0.50751922403943,0.856439875998617,
2.16199265283096));
#22038=CARTESIAN_POINT('Ctrl Pts',(-0.668734590074648,0.843674189185456,
2.15414210179328));
#22039=CARTESIAN_POINT('Ctrl Pts',(-0.768307141682156,0.971105204964537,
2.14629155075561));
#22040=CARTESIAN_POINT('Ctrl Pts',(-0.716937847311012,1.12444976178997,
2.13844099971793));
#22041=CARTESIAN_POINT('Ctrl Pts',(-0.560695911521528,1.16618480983832,
2.13059044868025));
#22042=CARTESIAN_POINT('Ctrl Pts',(-0.439702816507024,1.05888137703287,
2.12273989764257));
#22043=CARTESIAN_POINT('Ctrl Pts',(-0.462468046837819,0.8987717108876,2.11488934660489));
#22044=CARTESIAN_POINT('Ctrl Pts',(-0.608575201728667,0.829446009653423,
2.10703879556722));
#22045=CARTESIAN_POINT('Ctrl Pts',(-0.746991913163515,0.913077125320336,
2.09918824452953));
#22046=CARTESIAN_POINT('Ctrl Pts',(-0.753582779750997,1.07466285215048,
2.09133769349186));
#22047=CARTESIAN_POINT('Ctrl Pts',(-0.622436963324253,1.16928894070762,
2.08348714245418));
#22048=CARTESIAN_POINT('Ctrl Pts',(-0.471169134783152,1.11209310987848,
2.07563659141651));
#22049=CARTESIAN_POINT('Ctrl Pts',(-0.435439908588715,0.954368673788424,
2.06778604037882));
#22050=CARTESIAN_POINT('Ctrl Pts',(-0.547292045972571,0.837569145222665,
2.05993548934115));
#22051=CARTESIAN_POINT('Ctrl Pts',(-0.706414005411818,0.866438228174611,
2.05208493830347));
#22052=CARTESIAN_POINT('Ctrl Pts',(-0.770101205975101,1.01509505045675,
2.04423438726579));
#22053=CARTESIAN_POINT('Ctrl Pts',(-0.681237893770622,1.15020176258845,
2.03638383622811));
#22054=CARTESIAN_POINT('Ctrl Pts',(-0.519517932367091,1.15062854349327,
2.02853328519044));
#22055=CARTESIAN_POINT('Ctrl Pts',(-0.429977328488155,1.01591976127225,
2.02068273415276));
#22056=CARTESIAN_POINT('Ctrl Pts',(-0.492914923533471,0.867028771893199,
2.01283218311508));
#22057=CARTESIAN_POINT('Ctrl Pts',(-0.651892817203601,0.837201675931786,
2.0049816320774));
#22058=CARTESIAN_POINT('Ctrl Pts',(-0.764329038309151,0.95375831308653,
1.99713108103972));
#22059=CARTESIAN_POINT('Ctrl Pts',(-0.741000605841356,1.05850455157603,
1.99189738034794));
#22060=CARTESIAN_POINT('Ctrl Pts',(-0.709879644719091,1.09463771598849,
1.98928053000205));
#22061=CARTESIAN_POINT('Ctrl Pts',(-0.635056132297313,0.868871797975679,
2.41071946999795));
#22062=CARTESIAN_POINT('Ctrl Pts',(-0.678176738438398,0.880399765646142,
2.40810261965206));
#22063=CARTESIAN_POINT('Ctrl Pts',(-0.751456736091222,0.949093418718895,
2.40286891896028));
#22064=CARTESIAN_POINT('Ctrl Pts',(-0.725983267276729,1.09851903383873,
2.3950183679226));
#22065=CARTESIAN_POINT('Ctrl Pts',(-0.587321089598503,1.15929635946738,
2.38716781688492));
#22066=CARTESIAN_POINT('Ctrl Pts',(-0.460131718190347,1.07735615867206,
2.37931726584724));
#22067=CARTESIAN_POINT('Ctrl Pts',(-0.458327757321973,0.925968792387711,
2.37146671480957));
#22068=CARTESIAN_POINT('Ctrl Pts',(-0.583605177065917,0.841011131332347,
2.36361616377189));
#22069=CARTESIAN_POINT('Ctrl Pts',(-0.72357245622037,0.898619763467331,
2.35576561273421));
#22070=CARTESIAN_POINT('Ctrl Pts',(-0.752723842712768,1.04715812112138,
2.34791506169653));
#22071=CARTESIAN_POINT('Ctrl Pts',(-0.644905383184573,1.15339910973961,
2.34006451065885));
#22072=CARTESIAN_POINT('Ctrl Pts',(-0.496816476117644,1.12207059575698,
2.33221395962118));
#22073=CARTESIAN_POINT('Ctrl Pts',(-0.441264106639905,0.981265014401455,
2.3243634085835));
#22074=CARTESIAN_POINT('Ctrl Pts',(-0.528070317959361,0.857262052296277,
2.31651285754582));
#22075=CARTESIAN_POINT('Ctrl Pts',(-0.679384545107962,0.861269549983572,
2.30866230650814));
#22076=CARTESIAN_POINT('Ctrl Pts',(-0.759504943560701,0.989693978841561,
2.30081175547046));
#22077=CARTESIAN_POINT('Ctrl Pts',(-0.696577456243827,1.12736100826881,
2.29296120443279));
#22078=CARTESIAN_POINT('Ctrl Pts',(-0.547037040896711,1.15080770050942,
2.28511065339511));
#22079=CARTESIAN_POINT('Ctrl Pts',(-0.444995050756889,1.03900643986939,
2.27726010235743));
#22080=CARTESIAN_POINT('Ctrl Pts',(-0.481965192089592,0.892223287733,2.26940955131975));
#22081=CARTESIAN_POINT('Ctrl Pts',(-0.624791751222149,0.842096847750981,
2.26155900028208));
#22082=CARTESIAN_POINT('Ctrl Pts',(-0.745384480530408,0.933581711514867,
2.2537084492444));
#22083=CARTESIAN_POINT('Ctrl Pts',(-0.735592950331409,1.08463207393244,
2.24585789820672));
#22084=CARTESIAN_POINT('Ctrl Pts',(-0.604198439271435,1.15978238118065,
2.23800734716904));
#22085=CARTESIAN_POINT('Ctrl Pts',(-0.469038667788838,1.09163604999709,
2.23015679613136));
#22086=CARTESIAN_POINT('Ctrl Pts',(-0.451328132598973,0.941308330848865,
2.22230624509368));
#22087=CARTESIAN_POINT('Ctrl Pts',(-0.56695006249535,0.843616695807582,
2.21445569405601));
#22088=CARTESIAN_POINT('Ctrl Pts',(-0.712211962098838,0.886173325824406,
2.20660514301833));
#22089=CARTESIAN_POINT('Ctrl Pts',(-0.756839506387522,1.0308124232748,2.19875459198065));
#22090=CARTESIAN_POINT('Ctrl Pts',(-0.660809652710606,1.14781820705317,
2.19090404094297));
#22091=CARTESIAN_POINT('Ctrl Pts',(-0.51024425681279,1.13225710850146,2.1830534899053));
#22092=CARTESIAN_POINT('Ctrl Pts',(-0.440173945225492,0.998084690937051,
2.17520293886762));
#22093=CARTESIAN_POINT('Ctrl Pts',(-0.513439439211253,0.865629967835047,
2.16735238782994));
#22094=CARTESIAN_POINT('Ctrl Pts',(-0.664334501961606,0.853681484510555,
2.15950183679226));
#22095=CARTESIAN_POINT('Ctrl Pts',(-0.757532853908686,0.972954923483646,
2.15165128575458));
#22096=CARTESIAN_POINT('Ctrl Pts',(-0.709451997299263,1.11648303183743,
2.1438007347169));
#22097=CARTESIAN_POINT('Ctrl Pts',(-0.563211987522275,1.15554638447572,
2.13595018367923));
#22098=CARTESIAN_POINT('Ctrl Pts',(-0.449964341757637,1.05511204856404,
2.12809963264155));
#22099=CARTESIAN_POINT('Ctrl Pts',(-0.471272241517894,0.905251903628159,
2.12024908160387));
#22100=CARTESIAN_POINT('Ctrl Pts',(-0.608026254784307,0.840364130860531,
2.11239853056619));
#22101=CARTESIAN_POINT('Ctrl Pts',(-0.737582133180516,0.918641547938033,
2.10454797952851));
#22102=CARTESIAN_POINT('Ctrl Pts',(-0.7437510812886,1.06988326260355,2.09669742849084));
#22103=CARTESIAN_POINT('Ctrl Pts',(-0.621000646973074,1.15845180245062,
2.08884687745316));
#22104=CARTESIAN_POINT('Ctrl Pts',(-0.479416323833351,1.10491739878753,
2.08099632641548));
#22105=CARTESIAN_POINT('Ctrl Pts',(-0.445974326577002,0.957289791901268,
2.0731457753778));
#22106=CARTESIAN_POINT('Ctrl Pts',(-0.550666178876061,0.847967258785586,
2.06529522434013));
#22107=CARTESIAN_POINT('Ctrl Pts',(-0.699601845773343,0.87498826919366,
2.05744467330245));
#22108=CARTESIAN_POINT('Ctrl Pts',(-0.759212070044963,1.01412873128603,
2.04959412226477));
#22109=CARTESIAN_POINT('Ctrl Pts',(-0.676037398789558,1.14058650207107,
2.04174357122709));
#22110=CARTESIAN_POINT('Ctrl Pts',(-0.524670042661485,1.14098596232722,
2.03389302018941));
#22111=CARTESIAN_POINT('Ctrl Pts',(-0.440861436985121,1.01490064771879,
2.02604246915174));
#22112=CARTESIAN_POINT('Ctrl Pts',(-0.49977004220855,0.875541008883831,
2.01819191811406));
#22113=CARTESIAN_POINT('Ctrl Pts',(-0.648570865797738,0.847623313273011,
2.01034136707638));
#22114=CARTESIAN_POINT('Ctrl Pts',(-0.753809411330851,0.956718503824468,
2.0024908160387));
#22115=CARTESIAN_POINT('Ctrl Pts',(-0.731974363173429,1.05475934582637,
1.99725711534692));
#22116=CARTESIAN_POINT('Ctrl Pts',(-0.702845629995664,1.08857942294107,
1.99464026500102));
#22117=CARTESIAN_POINT('Ctrl Pts',(-0.632658506353108,0.877840168374445,
2.41607920499693));
#22118=CARTESIAN_POINT('Ctrl Pts',(-0.672829925654731,0.888579693265874,
2.41346235465104));
#22119=CARTESIAN_POINT('Ctrl Pts',(-0.74109801777064,0.952575118838442,
2.40822865395925));
#22120=CARTESIAN_POINT('Ctrl Pts',(-0.717366779080126,1.09178093194185,
2.40037810292158));
#22121=CARTESIAN_POINT('Ctrl Pts',(-0.588188249850668,1.1484014586541,2.3925275518839));
#22122=CARTESIAN_POINT('Ctrl Pts',(-0.469697856816082,1.07206546854677,
2.38467700084622));
#22123=CARTESIAN_POINT('Ctrl Pts',(-0.468017275884308,0.931032076110704,
2.37682644980854));
#22124=CARTESIAN_POINT('Ctrl Pts',(-0.584726483104016,0.851885001647656,
2.36897589877086));
#22125=CARTESIAN_POINT('Ctrl Pts',(-0.715120852817283,0.905553554202683,
2.36112534773319));
#22126=CARTESIAN_POINT('Ctrl Pts',(-0.742278462016426,1.04393279284724,
2.35327479669551));
#22127=CARTESIAN_POINT('Ctrl Pts',(-0.641834128465295,1.14290754489126,
2.34542424565783));
#22128=CARTESIAN_POINT('Ctrl Pts',(-0.50387360072502,1.1137217104627,2.33757369462015));
#22129=CARTESIAN_POINT('Ctrl Pts',(-0.452120674984892,0.98254637331334,
2.32972314358248));
#22130=CARTESIAN_POINT('Ctrl Pts',(-0.532989870132326,0.867024458591828,
2.32187259254479));
#22131=CARTESIAN_POINT('Ctrl Pts',(-0.673955125704091,0.870757867844471,
2.31402204150712));
#22132=CARTESIAN_POINT('Ctrl Pts',(-0.748595776865795,0.990398847921281,
2.30617149046944));
#22133=CARTESIAN_POINT('Ctrl Pts',(-0.689972146429509,1.11865029097931,
2.29832093943176));
#22134=CARTESIAN_POINT('Ctrl Pts',(-0.550659384735185,1.14049337226976,
2.29047038839408));
#22135=CARTESIAN_POINT('Ctrl Pts',(-0.455596445247116,1.0363386369461,2.28261983735641));
#22136=CARTESIAN_POINT('Ctrl Pts',(-0.490038054074624,0.899594558451655,
2.27476928631873));
#22137=CARTESIAN_POINT('Ctrl Pts',(-0.623096146429573,0.852896461675674,
2.26691873528105));
#22138=CARTESIAN_POINT('Ctrl Pts',(-0.735441067507883,0.938124317935081,
2.25906818424337));
#22139=CARTESIAN_POINT('Ctrl Pts',(-0.726319218340423,1.07884375551639,
2.25121763320569));
#22140=CARTESIAN_POINT('Ctrl Pts',(-0.603911291595331,1.14885423944223,
2.24336708216802));
#22141=CARTESIAN_POINT('Ctrl Pts',(-0.477995625308683,1.08536870227504,
2.23551653113034));
#22142=CARTESIAN_POINT('Ctrl Pts',(-0.461496382862034,0.945322483564629,
2.22766598009266));
#22143=CARTESIAN_POINT('Ctrl Pts',(-0.569210476934212,0.854312361381646,
2.21981542905498));
#22144=CARTESIAN_POINT('Ctrl Pts',(-0.704537347304013,0.893958377091083,
2.21196487801731));
#22145=CARTESIAN_POINT('Ctrl Pts',(-0.746112639361755,1.02870504118196,
2.20411432697963));
#22146=CARTESIAN_POINT('Ctrl Pts',(-0.656650642818685,1.1377083419588,2.19626377594195));
#22147=CARTESIAN_POINT('Ctrl Pts',(-0.516383003000816,1.12321152777512,
2.18841322490427));
#22148=CARTESIAN_POINT('Ctrl Pts',(-0.451105073971734,0.998215686412011,
2.18056267386659));
#22149=CARTESIAN_POINT('Ctrl Pts',(-0.519359654383078,0.874820059671476,
2.17271212282892));
#22150=CARTESIAN_POINT('Ctrl Pts',(-0.659934413848564,0.863688779835656,
2.16486157179123));
#22151=CARTESIAN_POINT('Ctrl Pts',(-0.746758566135216,0.974804642002754,
2.15701102075356));
#22152=CARTESIAN_POINT('Ctrl Pts',(-0.701966147287513,1.1085163018849,2.14916046971588));
#22153=CARTESIAN_POINT('Ctrl Pts',(-0.565728063523024,1.14490795911313,
2.1413099186782));
#22154=CARTESIAN_POINT('Ctrl Pts',(-0.46022586700825,1.0513427200952,2.13345936764053));
#22155=CARTESIAN_POINT('Ctrl Pts',(-0.48007643619797,0.91173209636872,2.12560881660285));
#22156=CARTESIAN_POINT('Ctrl Pts',(-0.607477307839948,0.851282252067638,
2.11775826556517));
#22157=CARTESIAN_POINT('Ctrl Pts',(-0.728172353197516,0.924205970555728,
2.10990771452749));
#22158=CARTESIAN_POINT('Ctrl Pts',(-0.733919382826205,1.06510367305662,
2.10205716348981));
#22159=CARTESIAN_POINT('Ctrl Pts',(-0.619564330621895,1.14761466419362,
2.09420661245214));
#22160=CARTESIAN_POINT('Ctrl Pts',(-0.487663512883551,1.09774168769659,
2.08635606141446));
#22161=CARTESIAN_POINT('Ctrl Pts',(-0.456508744565289,0.960210910014111,
2.07850551037678));
#22162=CARTESIAN_POINT('Ctrl Pts',(-0.554040311779553,0.858365372348507,
2.0706549593391));
#22163=CARTESIAN_POINT('Ctrl Pts',(-0.692789686134866,0.883538310212708,
2.06280440830143));
#22164=CARTESIAN_POINT('Ctrl Pts',(-0.748322934114825,1.01316241211532,
2.05495385726374));
#22165=CARTESIAN_POINT('Ctrl Pts',(-0.670836903808495,1.13097124155368,
2.04710330622607));
#22166=CARTESIAN_POINT('Ctrl Pts',(-0.529822152955879,1.13134338116118,
2.03925275518839));
#22167=CARTESIAN_POINT('Ctrl Pts',(-0.451745545482087,1.01388153416533,
2.03140220415071));
#22168=CARTESIAN_POINT('Ctrl Pts',(-0.506625160883627,0.884053245874464,
2.02355165311303));
#22169=CARTESIAN_POINT('Ctrl Pts',(-0.645248914391877,0.858044950614234,
2.01570110207536));
#22170=CARTESIAN_POINT('Ctrl Pts',(-0.743289784352549,0.959678694562408,
2.00785055103768));
#22171=CARTESIAN_POINT('Ctrl Pts',(-0.722948120505502,1.0510141400767,2.00261685034589));
#22172=CARTESIAN_POINT('Ctrl Pts',(-0.695811615272238,1.08252112989365,
2.));
#22173=CARTESIAN_POINT('Ctrl Pts',(-0.695811615272238,1.08252112989365,
2.));
#22174=CARTESIAN_POINT('Ctrl Pts',(-0.702493043757975,1.07628156364939,
2.));
#22175=CARTESIAN_POINT('Ctrl Pts',(-0.708395726655653,1.06931034161853,
2.));
#22176=CARTESIAN_POINT('Ctrl Pts',(-0.713512684042454,1.06178682515746,
2.));
#22177=CARTESIAN_POINT('Ctrl Pts',(-0.717502373507965,1.05592074262065,
2.));
#22178=CARTESIAN_POINT('Ctrl Pts',(-0.721014109525759,1.04971755287119,
2.));
#22179=CARTESIAN_POINT('Ctrl Pts',(-0.724031985841351,1.04324617113496,
2.));
#22180=CARTESIAN_POINT('Ctrl Pts',(-0.72532920883522,1.04046447158453,2.));
#22181=CARTESIAN_POINT('Ctrl Pts',(-0.726532666614568,1.03763771042115,
2.));
#22182=CARTESIAN_POINT('Ctrl Pts',(-0.727638826408048,1.0347790826819,2.));
#22183=CARTESIAN_POINT('Ctrl Pts',(-0.731193005346523,1.0255940855742,2.));
#22184=CARTESIAN_POINT('Ctrl Pts',(-0.733756270098347,1.01606060371262,
2.));
#22185=CARTESIAN_POINT('Ctrl Pts',(-0.73529467500939,1.0063604242084,2.));
#22186=CARTESIAN_POINT('Ctrl Pts',(-0.736007760405585,1.00186417208695,
2.));
#22187=CARTESIAN_POINT('Ctrl Pts',(-0.736500058162718,0.997331645993815,
2.));
#22188=CARTESIAN_POINT('Ctrl Pts',(-0.736764718140032,0.992779414308968,
2.));
#22189=CARTESIAN_POINT('Ctrl Pts',(-0.736959136386439,0.989435361647935,
2.));
#22190=CARTESIAN_POINT('Ctrl Pts',(-0.737030047799371,0.986088140051384,
2.));
#22191=CARTESIAN_POINT('Ctrl Pts',(-0.736976193579456,0.982751455795261,
2.));
#22192=CARTESIAN_POINT('Ctrl Pts',(-0.73686292459887,0.975733568899372,
2.));
#22193=CARTESIAN_POINT('Ctrl Pts',(-0.736199092496592,0.968753171717965,
2.));
#22194=CARTESIAN_POINT('Ctrl Pts',(-0.734968654150234,0.961871622922131,
2.));
#22195=CARTESIAN_POINT('Ctrl Pts',(-0.733610341240648,0.954274902131536,
2.));
#22196=CARTESIAN_POINT('Ctrl Pts',(-0.731561985767923,0.946798189069373,
2.));
#22197=CARTESIAN_POINT('Ctrl Pts',(-0.728883458720402,0.939498582185105,
2.));
#22198=CARTESIAN_POINT('Ctrl Pts',(-0.727748853408495,0.936406519794552,
2.));
#22199=CARTESIAN_POINT('Ctrl Pts',(-0.726503727419379,0.933354179904992,
2.));
#22200=CARTESIAN_POINT('Ctrl Pts',(-0.725155499563838,0.930349726147835,
2.));
#22201=CARTESIAN_POINT('Ctrl Pts',(-0.721333577255107,0.921832776440231,
2.));
#22202=CARTESIAN_POINT('Ctrl Pts',(-0.716682008196949,0.913689860477865,
2.));
#22203=CARTESIAN_POINT('Ctrl Pts',(-0.711310122504209,0.906016289602163,
2.));
#22204=CARTESIAN_POINT('Ctrl Pts',(-0.708434363463016,0.901908357660524,
2.));
#22205=CARTESIAN_POINT('Ctrl Pts',(-0.705351534711708,0.897934993684464,
2.));
#22206=CARTESIAN_POINT('Ctrl Pts',(-0.702074554712817,0.894112147617013,
2.));
#22207=CARTESIAN_POINT('Ctrl Pts',(-0.699663476442214,0.891299441684046,
2.));
#22208=CARTESIAN_POINT('Ctrl Pts',(-0.69714655627776,0.888568031452597,
2.));
#22209=CARTESIAN_POINT('Ctrl Pts',(-0.694540241228364,0.885935594383534,
2.));
#22210=CARTESIAN_POINT('Ctrl Pts',(-0.68996701323731,0.881316530816482,
2.));
#22211=CARTESIAN_POINT('Ctrl Pts',(-0.685111619991385,0.87699300942471,
2.));
#22212=CARTESIAN_POINT('Ctrl Pts',(-0.680004202609246,0.872997619450478,
2.));
#22213=CARTESIAN_POINT('Ctrl Pts',(-0.67522861092298,0.869261807450647,
2.));
#22214=CARTESIAN_POINT('Ctrl Pts',(-0.670227038735164,0.865810222770729,
2.));
#22215=CARTESIAN_POINT('Ctrl Pts',(-0.66504978274748,0.862688963354369,
2.));
#22216=CARTESIAN_POINT('Ctrl Pts',(-0.659173901912074,0.859146517620461,
2.));
#22217=CARTESIAN_POINT('Ctrl Pts',(-0.653067296294555,0.856024686886556,
2.));
#22218=CARTESIAN_POINT('Ctrl Pts',(-0.64676194038029,0.853364152629858,
2.));
#22219=CARTESIAN_POINT('Ctrl Pts',(-0.644516589878667,0.85241673078578,
2.));
#22220=CARTESIAN_POINT('Ctrl Pts',(-0.642245983976318,0.851527865406908,
2.));
#22221=CARTESIAN_POINT('Ctrl Pts',(-0.639952236162157,0.850696980524378,
2.));
#22222=CARTESIAN_POINT('Ctrl Pts',(-0.726369333664333,1.00010094057762,
2.35565803263806));
#22223=CARTESIAN_POINT('Ctrl Pts',(-0.726467565903334,1.01274184217687,
2.35486362065721));
#22224=CARTESIAN_POINT('Ctrl Pts',(-0.724719482090242,1.02535623071191,
2.35406920867636));
#22225=CARTESIAN_POINT('Ctrl Pts',(-0.721011471558047,1.03736537841382,
2.35327479669551));
#22226=CARTESIAN_POINT('Ctrl Pts',(-0.708797017499383,1.07692437686191,
2.35065794634961));
#22227=CARTESIAN_POINT('Ctrl Pts',(-0.675315572982339,1.10991596087659,
2.34804109600372));
#22228=CARTESIAN_POINT('Ctrl Pts',(-0.635581429433771,1.12154744714583,
2.34542424565783));
#22229=CARTESIAN_POINT('Ctrl Pts',(-0.595847285885203,1.13317893341507,
2.34280739531194));
#22230=CARTESIAN_POINT('Ctrl Pts',(-0.549860443305111,1.12345032193889,
2.34019054496604));
#22231=CARTESIAN_POINT('Ctrl Pts',(-0.518241534391711,1.09672346000923,
2.33757369462015));
#22232=CARTESIAN_POINT('Ctrl Pts',(-0.486622625478311,1.06999659807958,
2.33495684427426));
#22233=CARTESIAN_POINT('Ctrl Pts',(-0.469371650231601,1.02627148569646,
2.33233999392837));
#22234=CARTESIAN_POINT('Ctrl Pts',(-0.474224361799485,0.985155277051315,
2.32972314358247));
#22235=CARTESIAN_POINT('Ctrl Pts',(-0.47907707336737,0.944039068406169,
2.32710629323658));
#22236=CARTESIAN_POINT('Ctrl Pts',(-0.506033471749848,0.905531763498998,
2.32448944289069));
#22237=CARTESIAN_POINT('Ctrl Pts',(-0.543005880203048,0.886900345920854,
2.3218725925448));
#22238=CARTESIAN_POINT('Ctrl Pts',(-0.579978288656248,0.868268928342709,
2.3192557421989));
#22239=CARTESIAN_POINT('Ctrl Pts',(-0.62696670718017,0.86951339809359,2.31663889185301));
#22240=CARTESIAN_POINT('Ctrl Pts',(-0.662901024969081,0.890075796315165,
2.31402204150712));
#22241=CARTESIAN_POINT('Ctrl Pts',(-0.698835342757992,0.910638194536741,
2.31140519116123));
#22242=CARTESIAN_POINT('Ctrl Pts',(-0.723715559811894,0.950518521229011,
2.30878834081533));
#22243=CARTESIAN_POINT('Ctrl Pts',(-0.72638506326613,0.991833925084817,
2.30617149046944));
#22244=CARTESIAN_POINT('Ctrl Pts',(-0.726559659603113,0.994536119817981,
2.30600033785898));
#22245=CARTESIAN_POINT('Ctrl Pts',(-0.726639245398498,0.997244453365998,
2.30582918524852));
#22246=CARTESIAN_POINT('Ctrl Pts',(-0.726626272216059,0.999953562434948,
2.30565803263806));
#22247=CARTESIAN_POINT('Ctrl Pts',(-0.639851384185722,0.850935057178148,
2.4));
#22248=CARTESIAN_POINT('Ctrl Pts',(-0.649880557039356,0.854599675659919,
2.4));
#22249=CARTESIAN_POINT('Ctrl Pts',(-0.659434997625568,0.85936263163469,
2.4));
#22250=CARTESIAN_POINT('Ctrl Pts',(-0.668403171068605,0.865074092345247,
2.4));
#22251=CARTESIAN_POINT('Ctrl Pts',(-0.672868373471587,0.86791779605496,
2.4));
#22252=CARTESIAN_POINT('Ctrl Pts',(-0.67718781684999,0.870997354370473,
2.4));
#22253=CARTESIAN_POINT('Ctrl Pts',(-0.681344478651501,0.874297577803816,
2.4));
#22254=CARTESIAN_POINT('Ctrl Pts',(-0.684149819111287,0.8765249060701,2.4));
#22255=CARTESIAN_POINT('Ctrl Pts',(-0.686880965099162,0.878852785859471,
2.4));
#22256=CARTESIAN_POINT('Ctrl Pts',(-0.689531958931665,0.88127688968642,
2.4));
#22257=CARTESIAN_POINT('Ctrl Pts',(-0.691903137355438,0.883445126602317,
2.4));
#22258=CARTESIAN_POINT('Ctrl Pts',(-0.694203487834536,0.885684268626149,
2.4));
#22259=CARTESIAN_POINT('Ctrl Pts',(-0.696428596284293,0.887989081198335,
2.4));
#22260=CARTESIAN_POINT('Ctrl Pts',(-0.703655665265446,0.895475026186606,
2.4));
#22261=CARTESIAN_POINT('Ctrl Pts',(-0.710097115492295,0.903656379805453,
2.4));
#22262=CARTESIAN_POINT('Ctrl Pts',(-0.715619698888934,0.91241311638882,
2.4));
#22263=CARTESIAN_POINT('Ctrl Pts',(-0.717914152011463,0.916051254584994,
2.4));
#22264=CARTESIAN_POINT('Ctrl Pts',(-0.720049438182606,0.919788953917886,
2.4));
#22265=CARTESIAN_POINT('Ctrl Pts',(-0.722013340315698,0.923618244020841,
2.4));
#22266=CARTESIAN_POINT('Ctrl Pts',(-0.723497106826098,0.926511347662634,
2.4));
#22267=CARTESIAN_POINT('Ctrl Pts',(-0.724882791677009,0.929457049049758,
2.4));
#22268=CARTESIAN_POINT('Ctrl Pts',(-0.726159625039968,0.932438198899027,
2.4));
#22269=CARTESIAN_POINT('Ctrl Pts',(-0.7293219265251,0.939821538706109,2.4));
#22270=CARTESIAN_POINT('Ctrl Pts',(-0.731828922840258,0.947441945091078,
2.4));
#22271=CARTESIAN_POINT('Ctrl Pts',(-0.733609784156052,0.955243638029731,
2.4));
#22272=CARTESIAN_POINT('Ctrl Pts',(-0.735247937517986,0.962420148296355,
2.4));
#22273=CARTESIAN_POINT('Ctrl Pts',(-0.736271216774028,0.969750560405923,
2.4));
#22274=CARTESIAN_POINT('Ctrl Pts',(-0.736691013623241,0.977159425155101,
2.4));
#22275=CARTESIAN_POINT('Ctrl Pts',(-0.736867157952635,0.980268141943398,
2.4));
#22276=CARTESIAN_POINT('Ctrl Pts',(-0.736936476729183,0.983387171734525,
2.4));
#22277=CARTESIAN_POINT('Ctrl Pts',(-0.736900577814768,0.986501043637764,
2.4));
#22278=CARTESIAN_POINT('Ctrl Pts',(-0.73680325432052,0.994942883710025,
2.4));
#22279=CARTESIAN_POINT('Ctrl Pts',(-0.735935887531182,1.00336876050526,
2.4));
#22280=CARTESIAN_POINT('Ctrl Pts',(-0.73432454218896,1.01166505164342,2.4));
#22281=CARTESIAN_POINT('Ctrl Pts',(-0.733128713302574,1.01782198419718,
2.4));
#22282=CARTESIAN_POINT('Ctrl Pts',(-0.731522518607655,1.02390757353733,
2.4));
#22283=CARTESIAN_POINT('Ctrl Pts',(-0.729508194962256,1.0298701636783,2.4));
#22284=CARTESIAN_POINT('Ctrl Pts',(-0.728322998806314,1.03337845735825,
2.4));
#22285=CARTESIAN_POINT('Ctrl Pts',(-0.726998704692332,1.03683671166907,
2.4));
#22286=CARTESIAN_POINT('Ctrl Pts',(-0.72553907497761,1.04022912662095,2.4));
#22287=CARTESIAN_POINT('Ctrl Pts',(-0.723248641788982,1.04555246288699,
2.4));
#22288=CARTESIAN_POINT('Ctrl Pts',(-0.720623684757818,1.05071851440316,
2.4));
#22289=CARTESIAN_POINT('Ctrl Pts',(-0.717666939943194,1.055684952745,2.4));
#22290=CARTESIAN_POINT('Ctrl Pts',(-0.715625486572472,1.05911397788213,
2.4));
#22291=CARTESIAN_POINT('Ctrl Pts',(-0.713425317203702,1.06244758415869,
2.4));
#22292=CARTESIAN_POINT('Ctrl Pts',(-0.711075718450412,1.06565920682025,
2.4));
#22293=CARTESIAN_POINT('Ctrl Pts',(-0.707783291943712,1.07015956313241,
2.4));
#22294=CARTESIAN_POINT('Ctrl Pts',(-0.704194030655052,1.07442716580257,
2.4));
#22295=CARTESIAN_POINT('Ctrl Pts',(-0.700309061659577,1.07842077162732,
2.4));
#22296=CARTESIAN_POINT('Ctrl Pts',(-0.69890728532317,1.07986174635546,2.4));
#22297=CARTESIAN_POINT('Ctrl Pts',(-0.697466969165074,1.08126698735129,
2.4));
#22298=CARTESIAN_POINT('Ctrl Pts',(-0.695989827719556,1.08263574823442,
2.4));
#22299=CARTESIAN_POINT('Origin',(0.,0.,2.));
#22300=CARTESIAN_POINT('',(-0.8,0.6,2.));
#22301=CARTESIAN_POINT('',(0.8,0.6,2.));
#22302=CARTESIAN_POINT('Origin',(0.,0.,2.));
#22303=CARTESIAN_POINT('',(-1.8,0.6,2.));
#22304=CARTESIAN_POINT('',(-1.8,0.6,2.));
#22305=CARTESIAN_POINT('',(-1.8,1.4,2.));
#22306=CARTESIAN_POINT('',(-1.8,1.4,2.));
#22307=CARTESIAN_POINT('',(1.8,1.4,2.));
#22308=CARTESIAN_POINT('',(1.8,1.4,2.));
#22309=CARTESIAN_POINT('',(1.8,0.6,2.));
#22310=CARTESIAN_POINT('',(1.8,0.6,2.));
#22311=CARTESIAN_POINT('',(-1.8,0.6,2.));
#22312=CARTESIAN_POINT('Ctrl Pts',(0.504188384727762,1.08252112989365,2.));
#22313=CARTESIAN_POINT('Ctrl Pts',(0.497506952411728,1.07628156007241,2.));
#22314=CARTESIAN_POINT('Ctrl Pts',(0.491604265140002,1.06931033514179,2.));
#22315=CARTESIAN_POINT('Ctrl Pts',(0.486487303479808,1.06178681610824,2.));
#22316=CARTESIAN_POINT('Ctrl Pts',(0.482497614326221,1.0559207369233,2.));
#22317=CARTESIAN_POINT('Ctrl Pts',(0.478985877807952,1.04971755133896,2.));
#22318=CARTESIAN_POINT('Ctrl Pts',(0.47596800043997,1.04324617422688,2.));
#22319=CARTESIAN_POINT('Ctrl Pts',(0.474670775798635,1.04046447410142,2.));
#22320=CARTESIAN_POINT('Ctrl Pts',(0.473467316455455,1.03763771239116,2.));
#22321=CARTESIAN_POINT('Ctrl Pts',(0.472361155190705,1.03477908408591,2.));
#22322=CARTESIAN_POINT('Ctrl Pts',(0.468806973334995,1.02559408983729,2.));
#22323=CARTESIAN_POINT('Ctrl Pts',(0.466243705645806,1.01606061108597,2.));
#22324=CARTESIAN_POINT('Ctrl Pts',(0.464705298489784,1.00636043426204,2.));
#22325=CARTESIAN_POINT('Ctrl Pts',(0.463992209982944,1.00186417033063,2.));
#22326=CARTESIAN_POINT('Ctrl Pts',(0.463499910544365,0.997331632125338,
2.));
#22327=CARTESIAN_POINT('Ctrl Pts',(0.463235250450622,0.992779388102766,
2.));
#22328=CARTESIAN_POINT('Ctrl Pts',(0.463040833672037,0.989435353096635,
2.));
#22329=CARTESIAN_POINT('Ctrl Pts',(0.46296992260639,0.986088149337579,2.));
#22330=CARTESIAN_POINT('Ctrl Pts',(0.46302377604218,0.982751482606387,2.));
#22331=CARTESIAN_POINT('Ctrl Pts',(0.463137043908312,0.975733599437203,
2.));
#22332=CARTESIAN_POINT('Ctrl Pts',(0.463800875129207,0.968753205425666,
2.));
#22333=CARTESIAN_POINT('Ctrl Pts',(0.465031313050322,0.961871658945486,
2.));
#22334=CARTESIAN_POINT('Ctrl Pts',(0.466389625771061,0.954274939141924,
2.));
#22335=CARTESIAN_POINT('Ctrl Pts',(0.468437981894213,0.946798226077515,
2.));
#22336=CARTESIAN_POINT('Ctrl Pts',(0.471116510174533,0.93949861845872,2.));
#22337=CARTESIAN_POINT('Ctrl Pts',(0.472251116178103,0.936406555295212,
2.));
#22338=CARTESIAN_POINT('Ctrl Pts',(0.473496242998671,0.933354214505235,
2.));
#22339=CARTESIAN_POINT('Ctrl Pts',(0.474844471797333,0.930349759755262,
2.));
#22340=CARTESIAN_POINT('Ctrl Pts',(0.478666396590115,0.921832807655503,
2.));
#22341=CARTESIAN_POINT('Ctrl Pts',(0.483317968956197,0.913689888494062,
2.));
#22342=CARTESIAN_POINT('Ctrl Pts',(0.488689858313544,0.906016314077791,
2.));
#22343=CARTESIAN_POINT('Ctrl Pts',(0.491565612706781,0.90190838968258,2.));
#22344=CARTESIAN_POINT('Ctrl Pts',(0.494648435962255,0.897935032536209,
2.));
#22345=CARTESIAN_POINT('Ctrl Pts',(0.497925409635587,0.894112192538158,
2.));
#22346=CARTESIAN_POINT('Ctrl Pts',(0.500336494700513,0.891299477715359,
2.));
#22347=CARTESIAN_POINT('Ctrl Pts',(0.502853422244813,0.888568058918467,
2.));
#22348=CARTESIAN_POINT('Ctrl Pts',(0.505459745106002,0.885935613780059,
2.));
#22349=CARTESIAN_POINT('Ctrl Pts',(0.510032972332535,0.881316550670653,
2.));
#22350=CARTESIAN_POINT('Ctrl Pts',(0.514888364383629,0.876993029350264,
2.));
#22351=CARTESIAN_POINT('Ctrl Pts',(0.519995780056594,0.872997639132679,
2.));
#22352=CARTESIAN_POINT('Ctrl Pts',(0.52477137880872,0.869261820127707,2.));
#22353=CARTESIAN_POINT('Ctrl Pts',(0.529772958435197,0.865810229192487,
2.));
#22354=CARTESIAN_POINT('Ctrl Pts',(0.534950221975527,0.862688964531106,
2.));
#22355=CARTESIAN_POINT('Ctrl Pts',(0.540826105312277,0.859146516504166,
2.));
#22356=CARTESIAN_POINT('Ctrl Pts',(0.546932713096854,0.856024683905292,
2.));
#22357=CARTESIAN_POINT('Ctrl Pts',(0.553238070670066,0.853364148387157,
2.));
#22358=CARTESIAN_POINT('Ctrl Pts',(0.55548342158471,0.852416726168872,2.));
#22359=CARTESIAN_POINT('Ctrl Pts',(0.55775402783163,0.851527860483116,2.));
#22360=CARTESIAN_POINT('Ctrl Pts',(0.560047775926793,0.850696975355778,
2.));
#22361=CARTESIAN_POINT('Ctrl Pts',(0.639851384185725,0.850935057178149,
2.));
#22362=CARTESIAN_POINT('Ctrl Pts',(0.649880550625801,0.854599673316433,
2.));
#22363=CARTESIAN_POINT('Ctrl Pts',(0.659434984589242,0.859362630571034,
2.));
#22364=CARTESIAN_POINT('Ctrl Pts',(0.668403151796856,0.865074094293816,
2.));
#22365=CARTESIAN_POINT('Ctrl Pts',(0.672868418174611,0.867917842223432,
2.));
#22366=CARTESIAN_POINT('Ctrl Pts',(0.677187921251714,0.870997452272092,
2.));
#22367=CARTESIAN_POINT('Ctrl Pts',(0.68134463777063,0.874297734044997,2.));
#22368=CARTESIAN_POINT('Ctrl Pts',(0.684149977150149,0.876525071506887,
2.));
#22369=CARTESIAN_POINT('Ctrl Pts',(0.686881121795098,0.878852960779101,
2.));
#22370=CARTESIAN_POINT('Ctrl Pts',(0.689532114008666,0.881277074288136,
2.));
#22371=CARTESIAN_POINT('Ctrl Pts',(0.691903244332041,0.883445277204446,
2.));
#22372=CARTESIAN_POINT('Ctrl Pts',(0.694203548662863,0.885684381973589,
2.));
#22373=CARTESIAN_POINT('Ctrl Pts',(0.696428614090338,0.88798915510679,2.));
#22374=CARTESIAN_POINT('Ctrl Pts',(0.703655681573731,0.895475115187732,
2.));
#22375=CARTESIAN_POINT('Ctrl Pts',(0.710097129721786,0.903656484453022,
2.));
#22376=CARTESIAN_POINT('Ctrl Pts',(0.715619710640267,0.912413235085866,
2.));
#22377=CARTESIAN_POINT('Ctrl Pts',(0.717914173550032,0.916051396270592,
2.));
#22378=CARTESIAN_POINT('Ctrl Pts',(0.720049467939456,0.919789119253813,
2.));
#22379=CARTESIAN_POINT('Ctrl Pts',(0.722013376555431,0.923618433392056,
2.));
#22380=CARTESIAN_POINT('Ctrl Pts',(0.723497129119939,0.926511518450447,
2.));
#22381=CARTESIAN_POINT('Ctrl Pts',(0.724882801444961,0.929457199976584,
2.));
#22382=CARTESIAN_POINT('Ctrl Pts',(0.726159624011702,0.932438329054375,
2.));
#22383=CARTESIAN_POINT('Ctrl Pts',(0.729321918563565,0.939821663659088,
2.));
#22384=CARTESIAN_POINT('Ctrl Pts',(0.731828910123054,0.947442062000798,
2.));
#22385=CARTESIAN_POINT('Ctrl Pts',(0.733609769329411,0.955243743262114,
2.));
#22386=CARTESIAN_POINT('Ctrl Pts',(0.735247922763181,0.962420251602462,
2.));
#22387=CARTESIAN_POINT('Ctrl Pts',(0.736271202825978,0.969750659080777,
2.));
#22388=CARTESIAN_POINT('Ctrl Pts',(0.736691001072906,0.977159517273332,
2.));
#22389=CARTESIAN_POINT('Ctrl Pts',(0.736867146035702,0.980268232138734,
2.));
#22390=CARTESIAN_POINT('Ctrl Pts',(0.736936465492878,0.983387259690693,
2.));
#22391=CARTESIAN_POINT('Ctrl Pts',(0.736900567292279,0.986501129084147,
2.));
#22392=CARTESIAN_POINT('Ctrl Pts',(0.736803245735092,0.994942962189629,
2.));
#22393=CARTESIAN_POINT('Ctrl Pts',(0.73593588116366,1.00336883005034,2.));
#22394=CARTESIAN_POINT('Ctrl Pts',(0.734324538110121,1.01166511142386,2.));
#22395=CARTESIAN_POINT('Ctrl Pts',(0.733128714763866,1.01782201695168,2.));
#22396=CARTESIAN_POINT('Ctrl Pts',(0.731522528281544,1.02390757926145,2.));
#22397=CARTESIAN_POINT('Ctrl Pts',(0.729508215420297,1.02987014335002,2.));
#22398=CARTESIAN_POINT('Ctrl Pts',(0.728323015262132,1.03337845233062,2.));
#22399=CARTESIAN_POINT('Ctrl Pts',(0.726998715515976,1.03683672165704,2.));
#22400=CARTESIAN_POINT('Ctrl Pts',(0.725539078662676,1.04022915093548,2.));
#22401=CARTESIAN_POINT('Ctrl Pts',(0.723248638897094,1.04555249893377,2.));
#22402=CARTESIAN_POINT('Ctrl Pts',(0.72062367285432,1.05071856137362,2.));
#22403=CARTESIAN_POINT('Ctrl Pts',(0.717666916538866,1.05568500977016,2.));
#22404=CARTESIAN_POINT('Ctrl Pts',(0.71562546757316,1.05911402111255,2.));
#22405=CARTESIAN_POINT('Ctrl Pts',(0.713425303385499,1.06244761425647,2.));
#22406=CARTESIAN_POINT('Ctrl Pts',(0.711075710473028,1.06565922484506,2.));
#22407=CARTESIAN_POINT('Ctrl Pts',(0.707783289804617,1.0701595674468,2.));
#22408=CARTESIAN_POINT('Ctrl Pts',(0.704194035235276,1.07442715810878,2.));
#22409=CARTESIAN_POINT('Ctrl Pts',(0.700309073757905,1.07842075422663,2.));
#22410=CARTESIAN_POINT('Ctrl Pts',(0.698907297616712,1.07986172804018,2.));
#22411=CARTESIAN_POINT('Ctrl Pts',(0.697466981619643,1.08126696829348,2.));
#22412=CARTESIAN_POINT('Ctrl Pts',(0.695989840302895,1.08263572859343,2.));
#22413=CARTESIAN_POINT('Origin',(0.6,1.,2.51042117235887));
#22414=CARTESIAN_POINT('Ctrl Pts',(0.445511859130131,1.0000741974826,2.38542117235887));
#22415=CARTESIAN_POINT('Ctrl Pts',(0.445481645904189,1.00486660347515,2.38517311518799));
#22416=CARTESIAN_POINT('Ctrl Pts',(0.447840382858598,1.06018738535655,2.38230820767121));
#22417=CARTESIAN_POINT('Ctrl Pts',(0.514365803623529,1.16027111832567,2.37682644980854));
#22418=CARTESIAN_POINT('Ctrl Pts',(0.686438402045863,1.1598170503231,2.36897589877086));
#22419=CARTESIAN_POINT('Ctrl Pts',(0.780990355889297,1.01606136385454,2.36112534773319));
#22420=CARTESIAN_POINT('Ctrl Pts',(0.713226176840859,0.857888178208998,
2.35327479669551));
#22421=CARTESIAN_POINT('Ctrl Pts',(0.54391790721615,0.827171013394288,2.34542424565783));
#22422=CARTESIAN_POINT('Ctrl Pts',(0.453699048722976,0.921380393628473,
2.33947303754562));
#22423=CARTESIAN_POINT('Ctrl Pts',(0.445641803334383,0.985947130304853,
2.3361386797793));
#22424=CARTESIAN_POINT('Ctrl Pts',(0.445758404806891,0.999869526120069,
2.33542117235887));
#22425=CARTESIAN_POINT('Ctrl Pts',(0.445864724392684,0.99983533609866,2.38957882764113));
#22426=CARTESIAN_POINT('Ctrl Pts',(0.446099244735942,1.0340318743782,2.38781885106897));
#22427=CARTESIAN_POINT('Ctrl Pts',(0.47398874803022,1.11953643095444,2.38344202415091));
#22428=CARTESIAN_POINT('Ctrl Pts',(0.614413228882944,1.18108612135922,2.37644834688697));
#22429=CARTESIAN_POINT('Ctrl Pts',(0.759000551270414,1.08793755388759,2.36859779584929));
#22430=CARTESIAN_POINT('Ctrl Pts',(0.761051274433651,0.91584221771742,2.36074724481161));
#22431=CARTESIAN_POINT('Ctrl Pts',(0.618637433005314,0.819263404514795,
2.35289669377393));
#22432=CARTESIAN_POINT('Ctrl Pts',(0.475625295654385,0.878125251073759,
2.34584055471711));
#22433=CARTESIAN_POINT('Ctrl Pts',(0.446073423867575,0.964737113217481,
2.34140126600617));
#22434=CARTESIAN_POINT('Ctrl Pts',(0.445798439227784,1.00012317213786,2.33957882764113));
#22435=CARTESIAN_POINT('Ctrl Pts',(0.695811615272236,1.08252112989365,2.4));
#22436=CARTESIAN_POINT('Ctrl Pts',(0.7229481205055,1.0510141400767,2.39738314965411));
#22437=CARTESIAN_POINT('Ctrl Pts',(0.743289653273766,0.959678556377187,
2.39214944896232));
#22438=CARTESIAN_POINT('Ctrl Pts',(0.645248987396393,0.85804501052042,2.38429889792465));
#22439=CARTESIAN_POINT('Ctrl Pts',(0.506625118128944,0.884053189554221,
2.37644834688697));
#22440=CARTESIAN_POINT('Ctrl Pts',(0.45174554898112,1.01388156392493,2.36859779584929));
#22441=CARTESIAN_POINT('Ctrl Pts',(0.529822137836651,1.13134337597071,2.36074724481161));
#22442=CARTESIAN_POINT('Ctrl Pts',(0.670836914703171,1.13097126385843,2.35289669377393));
#22443=CARTESIAN_POINT('Ctrl Pts',(0.748322945574864,1.01316240738436,2.34504614273625));
#22444=CARTESIAN_POINT('Ctrl Pts',(0.692789695797321,0.883538302880933,
2.33719559169858));
#22445=CARTESIAN_POINT('Ctrl Pts',(0.554040306983033,0.858365357379829,
2.3293450406609));
#22446=CARTESIAN_POINT('Ctrl Pts',(0.456508731628746,0.960210907421746,
2.32149448962322));
#22447=CARTESIAN_POINT('Ctrl Pts',(0.487663502390397,1.09774169610628,2.31364393858554));
#22448=CARTESIAN_POINT('Ctrl Pts',(0.619564332496711,1.14761467812196,2.30579338754787));
#22449=CARTESIAN_POINT('Ctrl Pts',(0.733919395128131,1.0651036788751,2.29794283651019));
#22450=CARTESIAN_POINT('Ctrl Pts',(0.728172365024857,0.924205963670542,
2.29009228547251));
#22451=CARTESIAN_POINT('Ctrl Pts',(0.607477308519567,0.851282238312653,
2.28224173443483));
#22452=CARTESIAN_POINT('Ctrl Pts',(0.480076425153724,0.911732088265042,
2.27439118339715));
#22453=CARTESIAN_POINT('Ctrl Pts',(0.46022585412805,1.05134272481009,2.26654063235948));
#22454=CARTESIAN_POINT('Ctrl Pts',(0.565728060366633,1.14490797247226,2.2586900813218));
#22455=CARTESIAN_POINT('Ctrl Pts',(0.701966156681371,1.1085163118784,2.25083953028412));
#22456=CARTESIAN_POINT('Ctrl Pts',(0.746758579656851,0.974804639683806,
2.24298897924644));
#22457=CARTESIAN_POINT('Ctrl Pts',(0.659934419370361,0.863688767275607,
2.23513842820876));
#22458=CARTESIAN_POINT('Ctrl Pts',(0.519359646953508,0.874820048138925,
2.22728787717109));
#22459=CARTESIAN_POINT('Ctrl Pts',(0.451105060253533,0.998215686247253,
2.21943732613341));
#22460=CARTESIAN_POINT('Ctrl Pts',(0.516382995296938,1.12321153912718,2.21158677509573));
#22461=CARTESIAN_POINT('Ctrl Pts',(0.656650648038066,1.13770835464619,2.20373622405805));
#22462=CARTESIAN_POINT('Ctrl Pts',(0.746112652823594,1.02870504382673,2.19588567302037));
#22463=CARTESIAN_POINT('Ctrl Pts',(0.704537356935342,0.893958367321059,
2.1880351219827));
#22464=CARTESIAN_POINT('Ctrl Pts',(0.569210474097529,0.854312347959086,
2.18018457094502));
#22465=CARTESIAN_POINT('Ctrl Pts',(0.461496370101168,0.945322478526838,
2.17233401990734));
#22466=CARTESIAN_POINT('Ctrl Pts',(0.477995614068202,1.08536871014064,2.16448346886966));
#22467=CARTESIAN_POINT('Ctrl Pts',(0.603911291955373,1.14885425315604,2.15663291783199));
#22468=CARTESIAN_POINT('Ctrl Pts',(0.726319229979197,1.07884376278165,2.14878236679431));
#22469=CARTESIAN_POINT('Ctrl Pts',(0.73544107998541,0.938124312232147,2.14093181575663));
#22470=CARTESIAN_POINT('Ctrl Pts',(0.623096148559508,0.852896448126576,
2.13308126471895));
#22471=CARTESIAN_POINT('Ctrl Pts',(0.490038043939787,0.899594549193445,
2.12523071368128));
#22472=CARTESIAN_POINT('Ctrl Pts',(0.455596431949525,1.03633864030821,2.11738016264359));
#22473=CARTESIAN_POINT('Ctrl Pts',(0.550659380176962,1.14049338518748,2.10952961160592));
#22474=CARTESIAN_POINT('Ctrl Pts',(0.689972154741195,1.11865030196008,2.10167906056824));
#22475=CARTESIAN_POINT('Ctrl Pts',(0.748595790516416,0.990398846945399,
2.09382850953056));
#22476=CARTESIAN_POINT('Ctrl Pts',(0.673955132588938,0.870757856106032,
2.08597795849288));
#22477=CARTESIAN_POINT('Ctrl Pts',(0.532989863833319,0.867024446028552,
2.0781274074552));
#22478=CARTESIAN_POINT('Ctrl Pts',(0.45212066157753,0.982546372277999,2.07027685641753));
#22479=CARTESIAN_POINT('Ctrl Pts',(0.503873591498137,1.11372171989345,2.06242630537985));
#22480=CARTESIAN_POINT('Ctrl Pts',(0.641834132936712,1.14290755996024,2.05457575434217));
#22481=CARTESIAN_POINT('Ctrl Pts',(0.742278474130153,1.04393279346011,2.04672520330449));
#22482=CARTESIAN_POINT('Ctrl Pts',(0.71512086495066,0.905553551654031,2.03887465226682));
#22483=CARTESIAN_POINT('Ctrl Pts',(0.584726479537104,0.851884977081971,
2.03102410122914));
#22484=CARTESIAN_POINT('Ctrl Pts',(0.468017266318098,0.931032088917713,
2.02317355019146));
#22485=CARTESIAN_POINT('Ctrl Pts',(0.469697842938816,1.07206544198931,2.01532299915378));
#22486=CARTESIAN_POINT('Ctrl Pts',(0.588188246262365,1.1484015292732,2.0074724481161));
#22487=CARTESIAN_POINT('Ctrl Pts',(0.717366805638866,1.09178084131602,1.99962189707843));
#22488=CARTESIAN_POINT('Ctrl Pts',(0.741097987339953,0.952575306856465,
1.99177134604075));
#22489=CARTESIAN_POINT('Ctrl Pts',(0.672829925654733,0.888579693265875,
1.98653764534896));
#22490=CARTESIAN_POINT('Ctrl Pts',(0.63265850635311,0.877840168374445,1.98392079500307));
#22491=CARTESIAN_POINT('Ctrl Pts',(0.702845629995662,1.08857942294107,2.40535973499898));
#22492=CARTESIAN_POINT('Ctrl Pts',(0.731974363173428,1.05475934582637,2.40274288465309));
#22493=CARTESIAN_POINT('Ctrl Pts',(0.753809270628911,0.956718355494374,
2.3975091839613));
#22494=CARTESIAN_POINT('Ctrl Pts',(0.648570944161886,0.84762337757721,2.38965863292362));
#22495=CARTESIAN_POINT('Ctrl Pts',(0.499769996315029,0.875540948428836,
2.38180808188594));
#22496=CARTESIAN_POINT('Ctrl Pts',(0.440861440741036,1.01490067966319,2.37395753084827));
#22497=CARTESIAN_POINT('Ctrl Pts',(0.524670026432277,1.1409859567557,2.36610697981059));
#22498=CARTESIAN_POINT('Ctrl Pts',(0.676037410484068,1.14058652601332,2.35825642877291));
#22499=CARTESIAN_POINT('Ctrl Pts',(0.759212082346341,1.01412872620776,2.35040587773524));
#22500=CARTESIAN_POINT('Ctrl Pts',(0.699601856145167,0.87498826132362,2.34255532669755));
#22501=CARTESIAN_POINT('Ctrl Pts',(0.550666173727406,0.847967242717983,
2.33470477565988));
#22502=CARTESIAN_POINT('Ctrl Pts',(0.445974312690722,0.957289789118585,
2.32685422462219));
#22503=CARTESIAN_POINT('Ctrl Pts',(0.479416312569843,1.10491740781463,2.31900367358452));
#22504=CARTESIAN_POINT('Ctrl Pts',(0.62100064898553,1.15845181740151,2.31115312254684));
#22505=CARTESIAN_POINT('Ctrl Pts',(0.743751094493674,1.06988326884919,2.30330257150917));
#22506=CARTESIAN_POINT('Ctrl Pts',(0.737582145876161,0.918641540547371,
2.29545202047149));
#22507=CARTESIAN_POINT('Ctrl Pts',(0.608026255513821,0.840364116095719,
2.28760146943381));
#22508=CARTESIAN_POINT('Ctrl Pts',(0.471272229662835,0.905251894929553,
2.27975091839613));
#22509=CARTESIAN_POINT('Ctrl Pts',(0.449964327931837,1.05511205362507,2.27190036735845));
#22510=CARTESIAN_POINT('Ctrl Pts',(0.563211984134157,1.15554639881562,2.26404981632078));
#22511=CARTESIAN_POINT('Ctrl Pts',(0.709452007382772,1.11648304256461,2.2561992652831));
#22512=CARTESIAN_POINT('Ctrl Pts',(0.757532868423012,0.972954920994454,
2.24834871424542));
#22513=CARTESIAN_POINT('Ctrl Pts',(0.664334507888787,0.853681471028408,
2.24049816320774));
#22514=CARTESIAN_POINT('Ctrl Pts',(0.513439431236242,0.865629955455834,
2.23264761217006));
#22515=CARTESIAN_POINT('Ctrl Pts',(0.440173930500167,0.998084690760198,
2.22479706113238));
#22516=CARTESIAN_POINT('Ctrl Pts',(0.510244248543333,1.13225712068693,2.21694651009471));
#22517=CARTESIAN_POINT('Ctrl Pts',(0.660809658313168,1.14781822067201,2.20909595905703));
#22518=CARTESIAN_POINT('Ctrl Pts',(0.756839520837664,1.03081242611373,2.20124540801935));
#22519=CARTESIAN_POINT('Ctrl Pts',(0.71221197243725,0.886173315337117,2.19339485698167));
#22520=CARTESIAN_POINT('Ctrl Pts',(0.566950059450412,0.843616681399604,
2.18554430594399));
#22521=CARTESIAN_POINT('Ctrl Pts',(0.451328118901268,0.941308325441225,
2.17769375490632));
#22522=CARTESIAN_POINT('Ctrl Pts',(0.469038655723137,1.09163605844015,2.16984320386864));
#22523=CARTESIAN_POINT('Ctrl Pts',(0.604198439657909,1.15978239590126,2.16199265283096));
#22524=CARTESIAN_POINT('Ctrl Pts',(0.735592962824645,1.08463208173108,2.15414210179328));
#22525=CARTESIAN_POINT('Ctrl Pts',(0.745384493923972,0.933581705393252,
2.14629155075561));
#22526=CARTESIAN_POINT('Ctrl Pts',(0.624791753508452,0.842096833207175,
2.13844099971793));
#22527=CARTESIAN_POINT('Ctrl Pts',(0.481965181210706,0.892223277795097,
2.13059044868025));
#22528=CARTESIAN_POINT('Ctrl Pts',(0.444995036483054,1.03900644347833,2.12273989764257));
#22529=CARTESIAN_POINT('Ctrl Pts',(0.547037036003845,1.15080771437549,2.11488934660489));
#22530=CARTESIAN_POINT('Ctrl Pts',(0.696577465165717,1.12736102005574,2.10703879556722));
#22531=CARTESIAN_POINT('Ctrl Pts',(0.759504958213481,0.989693977794033,
2.09918824452954));
#22532=CARTESIAN_POINT('Ctrl Pts',(0.679384552498262,0.861269537383356,
2.09133769349186));
#22533=CARTESIAN_POINT('Ctrl Pts',(0.52807031119791,0.857262038810666,2.08348714245418));
#22534=CARTESIAN_POINT('Ctrl Pts',(0.441264092248243,0.981265013290105,
2.07563659141651));
#22535=CARTESIAN_POINT('Ctrl Pts',(0.496816466213367,1.12207060588009,2.06778604037882));
#22536=CARTESIAN_POINT('Ctrl Pts',(0.644905387984261,1.15339912591488,2.05993548934115));
#22537=CARTESIAN_POINT('Ctrl Pts',(0.752723855715824,1.04715812177925,2.05208493830347));
#22538=CARTESIAN_POINT('Ctrl Pts',(0.723572469244521,0.89861976073157,2.04423438726579));
#22539=CARTESIAN_POINT('Ctrl Pts',(0.583605173237138,0.84101110496317,2.03638383622811));
#22540=CARTESIAN_POINT('Ctrl Pts',(0.458327747053459,0.92596880613495,2.02853328519044));
#22541=CARTESIAN_POINT('Ctrl Pts',(0.460131703294282,1.07735613016487,2.02068273415276));
#22542=CARTESIAN_POINT('Ctrl Pts',(0.587321085746765,1.15929643527098,2.01283218311508));
#22543=CARTESIAN_POINT('Ctrl Pts',(0.72598329578528,1.09851893655959,2.0049816320774));
#22544=CARTESIAN_POINT('Ctrl Pts',(0.751456703426463,0.949093620540274,
1.99713108103973));
#22545=CARTESIAN_POINT('Ctrl Pts',(0.6781767384384,0.880399765646143,1.99189738034794));
#22546=CARTESIAN_POINT('Ctrl Pts',(0.635056132297315,0.86887179797568,1.98928053000205));
#22547=CARTESIAN_POINT('Ctrl Pts',(0.709879644719089,1.09463771598849,2.41071946999795));
#22548=CARTESIAN_POINT('Ctrl Pts',(0.741000605841355,1.05850455157604,2.40810261965206));
#22549=CARTESIAN_POINT('Ctrl Pts',(0.764328887984058,0.953758154611561,
2.40286891896028));
#22550=CARTESIAN_POINT('Ctrl Pts',(0.651892900927377,0.837201744634001,
2.3950183679226));
#22551=CARTESIAN_POINT('Ctrl Pts',(0.492914874501113,0.867028707303451,
2.38716781688492));
#22552=CARTESIAN_POINT('Ctrl Pts',(0.429977332500953,1.01591979540145,2.37931726584724));
#22553=CARTESIAN_POINT('Ctrl Pts',(0.519517915027903,1.15062853754068,2.37146671480957));
#22554=CARTESIAN_POINT('Ctrl Pts',(0.681237906264966,1.15020178816821,2.36361616377189));
#22555=CARTESIAN_POINT('Ctrl Pts',(0.770101219117818,1.01509504503115,2.35576561273421));
#22556=CARTESIAN_POINT('Ctrl Pts',(0.706414016493014,0.866438219766308,
2.34791506169653));
#22557=CARTESIAN_POINT('Ctrl Pts',(0.547292040471776,0.837569128056136,
2.34006451065885));
#22558=CARTESIAN_POINT('Ctrl Pts',(0.435439893752698,0.954368670815423,
2.33221395962117));
#22559=CARTESIAN_POINT('Ctrl Pts',(0.471169122749288,1.11209311952297,2.3243634085835));
#22560=CARTESIAN_POINT('Ctrl Pts',(0.622436965474348,1.16928895668105,2.31651285754582));
#22561=CARTESIAN_POINT('Ctrl Pts',(0.753582793859216,1.07466285882328,2.30866230650814));
#22562=CARTESIAN_POINT('Ctrl Pts',(0.746991926727465,0.913077117424199,
2.30081175547046));
#22563=CARTESIAN_POINT('Ctrl Pts',(0.608575202508074,0.829445993878789,
2.29296120443279));
#22564=CARTESIAN_POINT('Ctrl Pts',(0.462468034171945,0.898771701594062,
2.28511065339511));
#22565=CARTESIAN_POINT('Ctrl Pts',(0.439702801735622,1.05888138244004,2.27726010235743));
#22566=CARTESIAN_POINT('Ctrl Pts',(0.560695907901683,1.16618482515898,2.26940955131976));
#22567=CARTESIAN_POINT('Ctrl Pts',(0.716937858084172,1.12444977325082,2.26155900028207));
#22568=CARTESIAN_POINT('Ctrl Pts',(0.768307157189173,0.9711052023051,2.2537084492444));
#22569=CARTESIAN_POINT('Ctrl Pts',(0.668734596407212,0.843674174781211,
2.24585789820672));
#22570=CARTESIAN_POINT('Ctrl Pts',(0.507519215518976,0.856439862772741,
2.23800734716904));
#22571=CARTESIAN_POINT('Ctrl Pts',(0.429242800746802,0.997953695273144,
2.23015679613136));
#22572=CARTESIAN_POINT('Ctrl Pts',(0.504105501789727,1.14130270224668,2.22230624509369));
#22573=CARTESIAN_POINT('Ctrl Pts',(0.664968668588271,1.15792808669784,2.214455694056));
#22574=CARTESIAN_POINT('Ctrl Pts',(0.767566388851732,1.03291980840074,2.20660514301833));
#22575=CARTESIAN_POINT('Ctrl Pts',(0.71988658793916,0.878388263353175,2.19875459198065));
#22576=CARTESIAN_POINT('Ctrl Pts',(0.564689644803295,0.832921014840122,
2.19090404094297));
#22577=CARTESIAN_POINT('Ctrl Pts',(0.441159867701366,0.937294172355611,
2.1830534899053));
#22578=CARTESIAN_POINT('Ctrl Pts',(0.460081697378071,1.09790340673965,2.17520293886761));
#22579=CARTESIAN_POINT('Ctrl Pts',(0.604485587360446,1.17071053864647,2.16735238782994));
#22580=CARTESIAN_POINT('Ctrl Pts',(0.744866695670093,1.09042040068052,2.15950183679226));
#22581=CARTESIAN_POINT('Ctrl Pts',(0.755327907862536,0.929039098554358,
2.15165128575458));
#22582=CARTESIAN_POINT('Ctrl Pts',(0.626487358457396,0.831297218287773,
2.1438007347169));
#22583=CARTESIAN_POINT('Ctrl Pts',(0.473892318481626,0.884852006396751,
2.13595018367923));
#22584=CARTESIAN_POINT('Ctrl Pts',(0.434393641016582,1.04167424664844,2.12809963264155));
#22585=CARTESIAN_POINT('Ctrl Pts',(0.54341469183073,1.1611220435635,2.12024908160387));
#22586=CARTESIAN_POINT('Ctrl Pts',(0.703182775590238,1.1360717381514,2.11239853056619));
#22587=CARTESIAN_POINT('Ctrl Pts',(0.770414125910549,0.988989108642668,
2.10454797952851));
#22588=CARTESIAN_POINT('Ctrl Pts',(0.684813972407585,0.851781218660681,
2.09669742849084));
#22589=CARTESIAN_POINT('Ctrl Pts',(0.523150758562502,0.84749963159278,2.08884687745316));
#22590=CARTESIAN_POINT('Ctrl Pts',(0.430407522918953,0.979983654302211,
2.08099632641548));
#22591=CARTESIAN_POINT('Ctrl Pts',(0.489759340928599,1.13041949186674,2.0731457753778));
#22592=CARTESIAN_POINT('Ctrl Pts',(0.647976643031809,1.16389069186952,2.06529522434013));
#22593=CARTESIAN_POINT('Ctrl Pts',(0.763169237301496,1.05038345009838,2.05744467330245));
#22594=CARTESIAN_POINT('Ctrl Pts',(0.732024073538381,0.89168596980911,2.04959412226477));
#22595=CARTESIAN_POINT('Ctrl Pts',(0.582483866937173,0.830137232844369,
2.04174357122709));
#22596=CARTESIAN_POINT('Ctrl Pts',(0.448638227788819,0.920905523352185,
2.03389302018941));
#22597=CARTESIAN_POINT('Ctrl Pts',(0.450565563649749,1.08264681834044,2.02604246915174));
#22598=CARTESIAN_POINT('Ctrl Pts',(0.586453925231163,1.17019134126876,2.01819191811406));
#22599=CARTESIAN_POINT('Ctrl Pts',(0.734599785931696,1.10525703180317,2.01034136707638));
#22600=CARTESIAN_POINT('Ctrl Pts',(0.761815419512973,0.945611934224082,
2.0024908160387));
#22601=CARTESIAN_POINT('Ctrl Pts',(0.683523551222068,0.872219838026411,
1.99725711534692));
#22602=CARTESIAN_POINT('Ctrl Pts',(0.63745375824152,0.859903427576914,1.99464026500102));
#22603=CARTESIAN_POINT('Ctrl Pts',(0.716913659442515,1.10069600903591,2.41607920499693));
#22604=CARTESIAN_POINT('Ctrl Pts',(0.750026848509282,1.0622497573257,2.41346235465104));
#22605=CARTESIAN_POINT('Ctrl Pts',(0.774848505339203,0.950797953728747,
2.40822865395925));
#22606=CARTESIAN_POINT('Ctrl Pts',(0.65521485769287,0.826780111690792,2.40037810292158));
#22607=CARTESIAN_POINT('Ctrl Pts',(0.486059752687198,0.858516466178065,
2.3925275518839));
#22608=CARTESIAN_POINT('Ctrl Pts',(0.419093224260869,1.01693891113971,2.38467700084622));
#22609=CARTESIAN_POINT('Ctrl Pts',(0.514365803623529,1.16027111832567,2.37682644980854));
#22610=CARTESIAN_POINT('Ctrl Pts',(0.686438402045863,1.1598170503231,2.36897589877086));
#22611=CARTESIAN_POINT('Ctrl Pts',(0.780990355889297,1.01606136385454,2.36112534773319));
#22612=CARTESIAN_POINT('Ctrl Pts',(0.713226176840859,0.857888178208998,
2.35327479669551));
#22613=CARTESIAN_POINT('Ctrl Pts',(0.54391790721615,0.827171013394288,2.34542424565783));
#22614=CARTESIAN_POINT('Ctrl Pts',(0.424905474814674,0.951447552512262,
2.33757369462016));
#22615=CARTESIAN_POINT('Ctrl Pts',(0.462921932928734,1.11926883123131,2.32972314358247));
#22616=CARTESIAN_POINT('Ctrl Pts',(0.623873281963166,1.1801260959606,2.3218725925448));
#22617=CARTESIAN_POINT('Ctrl Pts',(0.76341449322476,1.07944244879737,2.31402204150712));
#22618=CARTESIAN_POINT('Ctrl Pts',(0.756401707578768,0.907512694301026,
2.30617149046944));
#22619=CARTESIAN_POINT('Ctrl Pts',(0.609124149502328,0.818527871661859,
2.29832093943176));
#22620=CARTESIAN_POINT('Ctrl Pts',(0.453663838681055,0.892291508258571,
2.29047038839408));
#22621=CARTESIAN_POINT('Ctrl Pts',(0.429441275539409,1.06265071125502,2.28261983735641));
#22622=CARTESIAN_POINT('Ctrl Pts',(0.558179831669208,1.17682325150234,2.27476928631873));
#22623=CARTESIAN_POINT('Ctrl Pts',(0.724423708785572,1.13241650393702,2.26691873528105));
#22624=CARTESIAN_POINT('Ctrl Pts',(0.779081445955335,0.969255483615749,
2.25906818424337));
#22625=CARTESIAN_POINT('Ctrl Pts',(0.673134684925636,0.833666878534013,
2.25121763320569));
#22626=CARTESIAN_POINT('Ctrl Pts',(0.50159899980171,0.84724977008965,2.24336708216802));
#22627=CARTESIAN_POINT('Ctrl Pts',(0.418311670993437,0.997822699786089,
2.23551653113034));
#22628=CARTESIAN_POINT('Ctrl Pts',(0.497966755036121,1.15034828380644,2.22766598009266));
#22629=CARTESIAN_POINT('Ctrl Pts',(0.669127678863374,1.16803795272366,2.21981542905498));
#22630=CARTESIAN_POINT('Ctrl Pts',(0.778293256865801,1.03502719068774,2.21196487801731));
#22631=CARTESIAN_POINT('Ctrl Pts',(0.727561203441069,0.870603211369231,
2.20411432697963));
#22632=CARTESIAN_POINT('Ctrl Pts',(0.562429230156179,0.822225348280642,
2.19626377594195));
#22633=CARTESIAN_POINT('Ctrl Pts',(0.430991616501465,0.933280019269996,
2.18841322490427));
#22634=CARTESIAN_POINT('Ctrl Pts',(0.451124739033006,1.10417075503916,2.18056267386659));
#22635=CARTESIAN_POINT('Ctrl Pts',(0.604772735062981,1.18163868139168,2.17271212282892));
#22636=CARTESIAN_POINT('Ctrl Pts',(0.754140428515542,1.09620871962996,2.16486157179123));
#22637=CARTESIAN_POINT('Ctrl Pts',(0.765271321801097,0.924496491715462,
2.15701102075356));
#22638=CARTESIAN_POINT('Ctrl Pts',(0.628182963406343,0.820497603368372,
2.14916046971588));
#22639=CARTESIAN_POINT('Ctrl Pts',(0.465819455752544,0.877480734998406,
2.1413099186782));
#22640=CARTESIAN_POINT('Ctrl Pts',(0.423792245550112,1.04434204981856,2.13345936764053));
#22641=CARTESIAN_POINT('Ctrl Pts',(0.539792347657613,1.17143637275151,2.12560881660284));
#22642=CARTESIAN_POINT('Ctrl Pts',(0.70978808601476,1.14478245624706,2.11775826556517));
#22643=CARTESIAN_POINT('Ctrl Pts',(0.781323293607615,0.988284239491303,
2.10990771452749));
#22644=CARTESIAN_POINT('Ctrl Pts',(0.690243392316909,0.842292899938004,
2.10205716348982));
#22645=CARTESIAN_POINT('Ctrl Pts',(0.518231205927094,0.837737224374896,
2.09420661245213));
#22646=CARTESIAN_POINT('Ctrl Pts',(0.419550953589664,0.978702295314315,
2.08635606141446));
#22647=CARTESIAN_POINT('Ctrl Pts',(0.482702215643831,1.13876837785338,2.07850551037678));
#22648=CARTESIAN_POINT('Ctrl Pts',(0.651047898079357,1.17438225782416,2.0706549593391));
#22649=CARTESIAN_POINT('Ctrl Pts',(0.773614618887169,1.05360877841752,2.06280440830142));
#22650=CARTESIAN_POINT('Ctrl Pts',(0.740475677832241,0.884752178886651,
2.05495385726374));
#22651=CARTESIAN_POINT('Ctrl Pts',(0.581362560637208,0.819263360725568,
2.04710330622607));
#22652=CARTESIAN_POINT('Ctrl Pts',(0.438948708524181,0.915842240569421,
2.03925275518839));
#22653=CARTESIAN_POINT('Ctrl Pts',(0.440999424005214,1.08793750651601,2.03140220415071));
#22654=CARTESIAN_POINT('Ctrl Pts',(0.585586764715563,1.18108624726655,2.02355165311303));
#22655=CARTESIAN_POINT('Ctrl Pts',(0.74321627607811,1.11199512704675,2.01570110207536));
#22656=CARTESIAN_POINT('Ctrl Pts',(0.772174135599484,0.94213024790789,2.00785055103768));
#22657=CARTESIAN_POINT('Ctrl Pts',(0.688870364005735,0.864039910406678,
2.00261685034589));
#22658=CARTESIAN_POINT('Ctrl Pts',(0.639851384185725,0.850935057178149,
2.));
#22659=CARTESIAN_POINT('Ctrl Pts',(0.695811615272236,1.08252112989365,2.4));
#22660=CARTESIAN_POINT('Ctrl Pts',(0.702493035444011,1.07628157141353,2.4));
#22661=CARTESIAN_POINT('Ctrl Pts',(0.708395708847424,1.0693103556765,2.4));
#22662=CARTESIAN_POINT('Ctrl Pts',(0.713512656958279,1.06178684479855,2.4));
#22663=CARTESIAN_POINT('Ctrl Pts',(0.717502347100726,1.05592075498562,2.4));
#22664=CARTESIAN_POINT('Ctrl Pts',(0.721014082031974,1.04971755619462,2.4));
#22665=CARTESIAN_POINT('Ctrl Pts',(0.724031956062882,1.04324616442023,2.4));
#22666=CARTESIAN_POINT('Ctrl Pts',(0.725329175480596,1.04046446611758,2.4));
#22667=CARTESIAN_POINT('Ctrl Pts',(0.726532629865294,1.03763770614082,2.4));
#22668=CARTESIAN_POINT('Ctrl Pts',(0.727638786465014,1.03477907962968,2.4));
#22669=CARTESIAN_POINT('Ctrl Pts',(0.731192959070153,1.02559407631572,2.4));
#22670=CARTESIAN_POINT('Ctrl Pts',(0.733756217444906,1.01606058770234,2.4));
#22671=CARTESIAN_POINT('Ctrl Pts',(0.735294617481607,1.0063604023791,2.4));
#22672=CARTESIAN_POINT('Ctrl Pts',(0.736007696124321,1.00186417589745,2.4));
#22673=CARTESIAN_POINT('Ctrl Pts',(0.736499990230692,0.997331676100057,
2.4));
#22674=CARTESIAN_POINT('Ctrl Pts',(0.736764649954775,0.992779471200463,
2.4));
#22675=CARTESIAN_POINT('Ctrl Pts',(0.736959071387571,0.989435380209583,
2.4));
#22676=CARTESIAN_POINT('Ctrl Pts',(0.737029983554064,0.98608811988667,2.4));
#22677=CARTESIAN_POINT('Ctrl Pts',(0.736976127631269,0.982751397582665,
2.4));
#22678=CARTESIAN_POINT('Ctrl Pts',(0.736862856230108,0.975733502594741,
2.4));
#22679=CARTESIAN_POINT('Ctrl Pts',(0.736199022212823,0.968753098529686,
2.4));
#22680=CARTESIAN_POINT('Ctrl Pts',(0.73496858294117,0.96187154470407,2.4));
#22681=CARTESIAN_POINT('Ctrl Pts',(0.733610269619415,0.954274821768571,
2.4));
#22682=CARTESIAN_POINT('Ctrl Pts',(0.731561915556015,0.946798108708432,
2.4));
#22683=CARTESIAN_POINT('Ctrl Pts',(0.728883391181877,0.939498503415491,
2.4));
#22684=CARTESIAN_POINT('Ctrl Pts',(0.727748787370213,0.936406442701396,
2.4));
#22685=CARTESIAN_POINT('Ctrl Pts',(0.726503663184753,0.933354104764928,
2.4));
#22686=CARTESIAN_POINT('Ctrl Pts',(0.725155437375267,0.93034965316141,2.4));
#22687=CARTESIAN_POINT('Ctrl Pts',(0.721333520454809,0.921832708641144,
2.4));
#22688=CARTESIAN_POINT('Ctrl Pts',(0.716681958573065,0.913689799617633,
2.4));
#22689=CARTESIAN_POINT('Ctrl Pts',(0.711310080831161,0.906016236422445,
2.4));
#22690=CARTESIAN_POINT('Ctrl Pts',(0.708434311712215,0.901908288116612,
2.4));
#22691=CARTESIAN_POINT('Ctrl Pts',(0.705351471044678,0.897934909331024,
2.4));
#22692=CARTESIAN_POINT('Ctrl Pts',(0.702074477330367,0.894112050103086,
2.4));
#22693=CARTESIAN_POINT('Ctrl Pts',(0.699663413790917,0.891299363444374,
2.4));
#22694=CARTESIAN_POINT('Ctrl Pts',(0.697146509627061,0.888567971784173,
2.4));
#22695=CARTESIAN_POINT('Ctrl Pts',(0.694540211514707,0.885935552211034,
2.4));
#22696=CARTESIAN_POINT('Ctrl Pts',(0.689966981858787,0.881316487645227,
2.4));
#22697=CARTESIAN_POINT('Ctrl Pts',(0.685111586013864,0.876992966093948,
2.4));
#22698=CARTESIAN_POINT('Ctrl Pts',(0.680004164916354,0.87299757664439,2.4));
#22699=CARTESIAN_POINT('Ctrl Pts',(0.67522858856925,0.869261779852135,2.4));
#22700=CARTESIAN_POINT('Ctrl Pts',(0.670227032530533,0.865810208752244,
2.4));
#22701=CARTESIAN_POINT('Ctrl Pts',(0.665049792940119,0.862688960723077,
2.4));
#22702=CARTESIAN_POINT('Ctrl Pts',(0.659173917535639,0.859146519967616,
2.4));
#22703=CARTESIAN_POINT('Ctrl Pts',(0.653067316624201,0.856024693283448,
2.4));
#22704=CARTESIAN_POINT('Ctrl Pts',(0.646761964313973,0.85336416176701,2.4));
#22705=CARTESIAN_POINT('Ctrl Pts',(0.644516614709207,0.852416740735641,
2.4));
#22706=CARTESIAN_POINT('Ctrl Pts',(0.642246009555221,0.851527876023459,
2.4));
#22707=CARTESIAN_POINT('Ctrl Pts',(0.63995226235153,0.850696991672974,2.4));
#22708=CARTESIAN_POINT('Ctrl Pts',(0.473597863174539,0.999893075682974,
2.31934196736194));
#22709=CARTESIAN_POINT('Ctrl Pts',(0.473502307398787,0.988483568548598,
2.32005947478237));
#22710=CARTESIAN_POINT('Ctrl Pts',(0.474923175284874,0.977097443610316,
2.3207769822028));
#22711=CARTESIAN_POINT('Ctrl Pts',(0.477956455981403,0.966158447195516,
2.32149448962322));
#22712=CARTESIAN_POINT('Ctrl Pts',(0.489019256746842,0.926262390741107,
2.32411133996911));
#22713=CARTESIAN_POINT('Ctrl Pts',(0.521529781864938,0.892313874060468,
2.32672819031501));
#22714=CARTESIAN_POINT('Ctrl Pts',(0.5609099425597,0.879535106636999,2.3293450406609));
#22715=CARTESIAN_POINT('Ctrl Pts',(0.600290103254463,0.86675633921353,2.33196189100679));
#22716=CARTESIAN_POINT('Ctrl Pts',(0.646539899525892,0.875147321047232,
2.33457874135269));
#22717=CARTESIAN_POINT('Ctrl Pts',(0.678920339291197,0.90094682938132,2.33719559169858));
#22718=CARTESIAN_POINT('Ctrl Pts',(0.711300779056502,0.926746337715409,
2.33981244204447));
#22719=CARTESIAN_POINT('Ctrl Pts',(0.729811862315683,0.969954372549885,
2.34242929239036));
#22720=CARTESIAN_POINT('Ctrl Pts',(0.726153065466658,1.01119319937947,2.34504614273626));
#22721=CARTESIAN_POINT('Ctrl Pts',(0.722494268617633,1.05243202620905,2.34766299308215));
#22722=CARTESIAN_POINT('Ctrl Pts',(0.696665591660402,1.09170164503374,2.35027984342804));
#22723=CARTESIAN_POINT('Ctrl Pts',(0.6602487903707,1.11139847313147,2.35289669377393));
#22724=CARTESIAN_POINT('Ctrl Pts',(0.623831989080998,1.13109530122919,2.35551354411983));
#22725=CARTESIAN_POINT('Ctrl Pts',(0.576827063458825,1.13121933859995,2.35813039446572));
#22726=CARTESIAN_POINT('Ctrl Pts',(0.540311835838483,1.11170438861103,2.36074724481161));
#22727=CARTESIAN_POINT('Ctrl Pts',(0.503796608218141,1.09218943862212,2.3633640951575));
#22728=CARTESIAN_POINT('Ctrl Pts',(0.477771078599631,1.05303550127352,2.3659809455034));
#22729=CARTESIAN_POINT('Ctrl Pts',(0.473904908648346,1.01182047020411,2.36859779584929));
#22730=CARTESIAN_POINT('Ctrl Pts',(0.473538425642629,1.00791360406595,2.36884585302017));
#22731=CARTESIAN_POINT('Ctrl Pts',(0.473371057191087,1.00398821781876,2.36909391019106));
#22732=CARTESIAN_POINT('Ctrl Pts',(0.473395817154925,1.00006080538999,2.36934196736194));
#22733=CARTESIAN_POINT('Ctrl Pts',(0.560148615814278,0.850935057178148,
2.4));
#22734=CARTESIAN_POINT('Ctrl Pts',(0.511129635994267,0.864039910406677,
2.39738314965411));
#22735=CARTESIAN_POINT('Ctrl Pts',(0.427825810157124,0.942129912787787,
2.39214944896232));
#22736=CARTESIAN_POINT('Ctrl Pts',(0.456783771264579,1.11199528864852,2.38429889792464));
#22737=CARTESIAN_POINT('Ctrl Pts',(0.614413228882944,1.18108612135922,2.37644834688697));
#22738=CARTESIAN_POINT('Ctrl Pts',(0.759000551270414,1.08793755388759,2.36859779584929));
#22739=CARTESIAN_POINT('Ctrl Pts',(0.761051274433651,0.91584221771742,2.36074724481161));
#22740=CARTESIAN_POINT('Ctrl Pts',(0.618637433005314,0.819263404514795,
2.35289669377393));
#22741=CARTESIAN_POINT('Ctrl Pts',(0.459524343787705,0.884752183415202,
2.34504614273626));
#22742=CARTESIAN_POINT('Ctrl Pts',(0.426385402694383,1.05360877733288,2.33719559169858));
#22743=CARTESIAN_POINT('Ctrl Pts',(0.548952109888326,1.17438223097154,2.3293450406609));
#22744=CARTESIAN_POINT('Ctrl Pts',(0.717297767916034,1.1387683610531,2.32149448962322));
#22745=CARTESIAN_POINT('Ctrl Pts',(0.780449022522885,0.978702297157564,
2.31364393858554));
#22746=CARTESIAN_POINT('Ctrl Pts',(0.681768782849741,0.837737246759644,
2.30579338754786));
#22747=CARTESIAN_POINT('Ctrl Pts',(0.509756619949943,0.842292920851884,
2.29794283651019));
#22748=CARTESIAN_POINT('Ctrl Pts',(0.418676730713559,0.988284241230286,
2.29009228547251));
#22749=CARTESIAN_POINT('Ctrl Pts',(0.490211928794195,1.14478243668251,2.28224173443483));
#22750=CARTESIAN_POINT('Ctrl Pts',(0.660207644220989,1.17143634973614,2.27439118339715));
#22751=CARTESIAN_POINT('Ctrl Pts',(0.776207730757634,1.04434204382826,2.26654063235948));
#22752=CARTESIAN_POINT('Ctrl Pts',(0.734180526190243,0.87748075149375,2.2586900813218));
#22753=CARTESIAN_POINT('Ctrl Pts',(0.571817040388558,0.820497627508739,
2.25083953028412));
#22754=CARTESIAN_POINT('Ctrl Pts',(0.434728700430063,0.92449650187637,2.24298897924644));
#22755=CARTESIAN_POINT('Ctrl Pts',(0.445859592221225,1.09620870668547,2.23513842820877));
#22756=CARTESIAN_POINT('Ctrl Pts',(0.595227265578502,1.18163865695784,2.22728787717108));
#22757=CARTESIAN_POINT('Ctrl Pts',(0.748875240939872,1.10417074102503,2.21943732613341));
#22758=CARTESIAN_POINT('Ctrl Pts',(0.769008360762544,0.933280028245809,
2.21158677509573));
#22759=CARTESIAN_POINT('Ctrl Pts',(0.637570764789711,0.822225372195567,
2.20373622405805));
#22760=CARTESIAN_POINT('Ctrl Pts',(0.472438813719035,0.870603228776448,
2.19588567302037));
#22761=CARTESIAN_POINT('Ctrl Pts',(0.421706767119107,1.03502718597557,2.1880351219827));
#22762=CARTESIAN_POINT('Ctrl Pts',(0.530872330435983,1.16803793011858,2.18018457094502));
#22763=CARTESIAN_POINT('Ctrl Pts',(0.702033231237909,1.1503482635805,2.17233401990734));
#22764=CARTESIAN_POINT('Ctrl Pts',(0.781688304564893,0.997822700079642,
2.16448346886966));
#22765=CARTESIAN_POINT('Ctrl Pts',(0.698400986961052,0.847249790637147,
2.15663291783198));
#22766=CARTESIAN_POINT('Ctrl Pts',(0.526865324912526,0.833666900912216,
2.14878236679431));
#22767=CARTESIAN_POINT('Ctrl Pts',(0.420918578136115,0.969255487747401,
2.14093181575663));
#22768=CARTESIAN_POINT('Ctrl Pts',(0.475576307951429,1.13241648613165,2.13308126471895));
#22769=CARTESIAN_POINT('Ctrl Pts',(0.641820162707069,1.17682322770038,2.12523071368128));
#22770=CARTESIAN_POINT('Ctrl Pts',(0.770558701511974,1.06265070285456,2.11738016264359));
#22771=CARTESIAN_POINT('Ctrl Pts',(0.746336141641471,0.892291522696776,
2.10952961160592));
#22772=CARTESIAN_POINT('Ctrl Pts',(0.590875851708506,0.818527896169216,
2.10167906056824));
#22773=CARTESIAN_POINT('Ctrl Pts',(0.443598313494032,0.907512706568079,
2.09382850953057));
#22774=CARTESIAN_POINT('Ctrl Pts',(0.436585528693405,1.07944243843108,2.08597795849288));
#22775=CARTESIAN_POINT('Ctrl Pts',(0.57612672137744,1.18012607114374,2.07812740745521));
#22776=CARTESIAN_POINT('Ctrl Pts',(0.737078048375186,1.11926881624917,2.07027685641753));
#22777=CARTESIAN_POINT('Ctrl Pts',(0.775094502137202,0.951447557128672,
2.06242630537985));
#22778=CARTESIAN_POINT('Ctrl Pts',(0.656082084236305,0.827171040068,2.05457575434217));
#22779=CARTESIAN_POINT('Ctrl Pts',(0.48677384037764,0.857888191265152,2.04672520330449));
#22780=CARTESIAN_POINT('Ctrl Pts',(0.419009664523655,1.01606137229499,2.03887465226682));
#22781=CARTESIAN_POINT('Ctrl Pts',(0.513561617374857,1.15981701056446,2.03102410122914));
#22782=CARTESIAN_POINT('Ctrl Pts',(0.685634169421134,1.1602711276025,2.02317355019146));
#22783=CARTESIAN_POINT('Ctrl Pts',(0.780906782004492,1.01693885807272,2.01532299915378));
#22784=CARTESIAN_POINT('Ctrl Pts',(0.713940171081941,0.858516566589665,
2.0074724481161));
#22785=CARTESIAN_POINT('Ctrl Pts',(0.544785272473601,0.826780004858426,
1.99962189707843));
#22786=CARTESIAN_POINT('Ctrl Pts',(0.425151261024703,0.95079820002532,1.99177134604075));
#22787=CARTESIAN_POINT('Ctrl Pts',(0.449973151490716,1.0622497573257,1.98653764534896));
#22788=CARTESIAN_POINT('Ctrl Pts',(0.483086340557483,1.10069600903591,1.98392079500307));
#22789=CARTESIAN_POINT('Ctrl Pts',(0.562546241758482,0.859903427576914,
2.40535973499898));
#22790=CARTESIAN_POINT('Ctrl Pts',(0.516476448777934,0.872219838026409,
2.40274288465309));
#22791=CARTESIAN_POINT('Ctrl Pts',(0.438184529507143,0.945611619266206,
2.3975091839613));
#22792=CARTESIAN_POINT('Ctrl Pts',(0.46540025856266,1.1052571836823,2.38965863292362));
#22793=CARTESIAN_POINT('Ctrl Pts',(0.613546068752483,1.17019122293655,2.38180808188594));
#22794=CARTESIAN_POINT('Ctrl Pts',(0.749434413113403,1.08264686286195,2.37395753084827));
#22795=CARTESIAN_POINT('Ctrl Pts',(0.751361756194339,0.920905501875057,
2.36610697981059));
#22796=CARTESIAN_POINT('Ctrl Pts',(0.617516127087842,0.830137273999053,
2.35825642877291));
#22797=CARTESIAN_POINT('Ctrl Pts',(0.467975946780819,0.891685974065206,
2.35040587773523));
#22798=CARTESIAN_POINT('Ctrl Pts',(0.436830782981619,1.050383449079,2.34255532669756));
#22799=CARTESIAN_POINT('Ctrl Pts',(0.552023364456505,1.16389066663247,2.33470477565987));
#22800=CARTESIAN_POINT('Ctrl Pts',(0.710240643620372,1.13041947607723,2.3268542246222));
#22801=CARTESIAN_POINT('Ctrl Pts',(0.769592454630765,0.979983656034563,
2.31900367358452));
#22802=CARTESIAN_POINT('Ctrl Pts',(0.676849230889565,0.847499652630768,
2.31115312254684));
#22803=CARTESIAN_POINT('Ctrl Pts',(0.515186039121242,0.851781238316293,
2.30330257150916));
#22804=CARTESIAN_POINT('Ctrl Pts',(0.429585896947362,0.988989110277028,
2.29545202047149));
#22805=CARTESIAN_POINT('Ctrl Pts',(0.496817238327747,1.13607171976393,2.28760146943381));
#22806=CARTESIAN_POINT('Ctrl Pts',(0.65658530053649,1.16112202193283,2.27975091839613));
#22807=CARTESIAN_POINT('Ctrl Pts',(0.765606336716589,1.04167424101854,2.27190036735845));
#22808=CARTESIAN_POINT('Ctrl Pts',(0.726107664547559,0.884852021899667,
2.26404981632077));
#22809=CARTESIAN_POINT('Ctrl Pts',(0.573512645109186,0.831297240975754,
2.2561992652831));
#22810=CARTESIAN_POINT('Ctrl Pts',(0.444672113031105,0.929039108103942,
2.24834871424542));
#22811=CARTESIAN_POINT('Ctrl Pts',(0.455133323819063,1.09042038851482,2.24049816320774));
#22812=CARTESIAN_POINT('Ctrl Pts',(0.595514413242444,1.17071051568267,2.23264761217006));
#22813=CARTESIAN_POINT('Ctrl Pts',(0.739918283799722,1.09790339356867,2.22479706113239));
#22814=CARTESIAN_POINT('Ctrl Pts',(0.758840110930535,0.9372941807914,2.21694651009471));
#22815=CARTESIAN_POINT('Ctrl Pts',(0.635310350446671,0.832921037316226,
2.20909595905703));
#22816=CARTESIAN_POINT('Ctrl Pts',(0.480113428188521,0.878388279713101,
2.20124540801935));
#22817=CARTESIAN_POINT('Ctrl Pts',(0.432433633690143,1.03291980397207,2.19339485698167));
#22818=CARTESIAN_POINT('Ctrl Pts',(0.535031340151599,1.15792806545277,2.185544305944));
#22819=CARTESIAN_POINT('Ctrl Pts',(0.695894485310114,1.14130268323763,2.17769375490632));
#22820=CARTESIAN_POINT('Ctrl Pts',(0.770757176282041,0.997953695549035,
2.16984320386864));
#22821=CARTESIAN_POINT('Ctrl Pts',(0.692480772040193,0.856439882084015,
2.16199265283096));
#22822=CARTESIAN_POINT('Ctrl Pts',(0.531265412839046,0.843674195813048,
2.15414210179328));
#22823=CARTESIAN_POINT('Ctrl Pts',(0.431692865452835,0.971105206188175,
2.1462915507556));
#22824=CARTESIAN_POINT('Ctrl Pts',(0.483062157645861,1.12444975651669,2.13844099971793));
#22825=CARTESIAN_POINT('Ctrl Pts',(0.639304086812941,1.16618480278905,2.13059044868025));
#22826=CARTESIAN_POINT('Ctrl Pts',(0.760297176696446,1.05888137454499,2.12273989764257));
#22827=CARTESIAN_POINT('Ctrl Pts',(0.73753194733446,0.898771715163604,2.11488934660489));
#22828=CARTESIAN_POINT('Ctrl Pts',(0.591424798629911,0.829446016911682,
2.10703879556722));
#22829=CARTESIAN_POINT('Ctrl Pts',(0.453008093077508,0.913077128953215,
2.09918824452954));
#22830=CARTESIAN_POINT('Ctrl Pts',(0.44641722674026,1.07466284908066,2.09133769349186));
#22831=CARTESIAN_POINT('Ctrl Pts',(0.577563037665274,1.16928893335727,2.08348714245418));
#22832=CARTESIAN_POINT('Ctrl Pts',(0.728830859679466,1.11209310544222,2.0756365914165));
#22833=CARTESIAN_POINT('Ctrl Pts',(0.76456008458585,0.954368675154091,2.06778604037883));
#22834=CARTESIAN_POINT('Ctrl Pts',(0.652707951494933,0.837569153125047,
2.05993548934115));
#22835=CARTESIAN_POINT('Ctrl Pts',(0.493585999689548,0.866438232036949,
2.05208493830347));
#22836=CARTESIAN_POINT('Ctrl Pts',(0.429898800067004,1.01509505296379,2.04423438726579));
#22837=CARTESIAN_POINT('Ctrl Pts',(0.518762111987321,1.15020175080161,2.03638383622811));
#22838=CARTESIAN_POINT('Ctrl Pts',(0.680482059638507,1.15062854625939,2.02853328519044));
#22839=CARTESIAN_POINT('Ctrl Pts',(0.770022673387457,1.01591974552719,2.02068273415276));
#22840=CARTESIAN_POINT('Ctrl Pts',(0.707085053854394,0.867028801673869,
2.01283218311508));
#22841=CARTESIAN_POINT('Ctrl Pts',(0.548107221407733,0.837201644229118,
2.0049816320774));
#22842=CARTESIAN_POINT('Ctrl Pts',(0.435670892436373,0.953758386089901,
1.99713108103972));
#22843=CARTESIAN_POINT('Ctrl Pts',(0.458999394158644,1.05850455157603,1.99189738034794));
#22844=CARTESIAN_POINT('Ctrl Pts',(0.490120355280909,1.09463771598849,1.98928053000205));
#22845=CARTESIAN_POINT('Ctrl Pts',(0.564943867702687,0.868871797975679,
2.41071946999795));
#22846=CARTESIAN_POINT('Ctrl Pts',(0.521823261561601,0.880399765646142,
2.40810261965206));
#22847=CARTESIAN_POINT('Ctrl Pts',(0.448543248857163,0.949093325744624,
2.40286891896027));
#22848=CARTESIAN_POINT('Ctrl Pts',(0.474016745860739,1.09851907871609,2.3950183679226));
#22849=CARTESIAN_POINT('Ctrl Pts',(0.612678908622024,1.15929632451388,2.38716781688491));
#22850=CARTESIAN_POINT('Ctrl Pts',(0.739868274956389,1.07735617183631,2.37931726584725));
#22851=CARTESIAN_POINT('Ctrl Pts',(0.741672237955028,0.925968786032693,
2.37146671480956));
#22852=CARTESIAN_POINT('Ctrl Pts',(0.616394821170369,0.841011143483312,
2.36361616377189));
#22853=CARTESIAN_POINT('Ctrl Pts',(0.476427549773933,0.898619764715207,
2.35576561273421));
#22854=CARTESIAN_POINT('Ctrl Pts',(0.447276163268855,1.04715812082513,2.34791506169653));
#22855=CARTESIAN_POINT('Ctrl Pts',(0.555094619024684,1.15339910229339,2.34006451065885));
#22856=CARTESIAN_POINT('Ctrl Pts',(0.703183519324712,1.12207059110137,2.33221395962117));
#22857=CARTESIAN_POINT('Ctrl Pts',(0.758735886738644,0.981265014911558,
2.3243634085835));
#22858=CARTESIAN_POINT('Ctrl Pts',(0.67192967892939,0.857262058501895,2.31651285754582));
#22859=CARTESIAN_POINT('Ctrl Pts',(0.52061545829254,0.861269555780702,2.30866230650814));
#22860=CARTESIAN_POINT('Ctrl Pts',(0.440495063181165,0.989693979323769,
2.30081175547046));
#22861=CARTESIAN_POINT('Ctrl Pts',(0.5034225478613,1.12736100284536,2.29296120443278));
#22862=CARTESIAN_POINT('Ctrl Pts',(0.652962956851991,1.15080769412952,2.28511065339511));
#22863=CARTESIAN_POINT('Ctrl Pts',(0.755004942675543,1.03900643820883,2.27726010235743));
#22864=CARTESIAN_POINT('Ctrl Pts',(0.718034802904875,0.892223292305585,
2.26940955131975));
#22865=CARTESIAN_POINT('Ctrl Pts',(0.575208249829814,0.84209685444277,2.26155900028207));
#22866=CARTESIAN_POINT('Ctrl Pts',(0.454615525632148,0.933581714331513,
2.25370844924439));
#22867=CARTESIAN_POINT('Ctrl Pts',(0.4644070554169,1.08463207034418,2.24585789820672));
#22868=CARTESIAN_POINT('Ctrl Pts',(0.595801560906386,1.1597823744075,2.23800734716904));
#22869=CARTESIAN_POINT('Ctrl Pts',(0.730961326659572,1.09163604611232,2.23015679613136));
#22870=CARTESIAN_POINT('Ctrl Pts',(0.748671861098526,0.941308333336992,
2.22230624509368));
#22871=CARTESIAN_POINT('Ctrl Pts',(0.63304993610363,0.843616702436886,2.214455694056));
#22872=CARTESIAN_POINT('Ctrl Pts',(0.487788042658006,0.886173330649751,
2.20660514301833));
#22873=CARTESIAN_POINT('Ctrl Pts',(0.443160500261181,1.03081242196857,2.19875459198065));
#22874=CARTESIAN_POINT('Ctrl Pts',(0.539190349867211,1.14781820078696,2.19090404094297));
#22875=CARTESIAN_POINT('Ctrl Pts',(0.689755739382323,1.13225710289476,2.18305348990529));
#22876=CARTESIAN_POINT('Ctrl Pts',(0.759826047999188,0.998084691018425,
2.17520293886762));
#22877=CARTESIAN_POINT('Ctrl Pts',(0.686560557119336,0.865629973530885,
2.16735238782994));
#22878=CARTESIAN_POINT('Ctrl Pts',(0.535665500765565,0.853681490713878,
2.15950183679226));
#22879=CARTESIAN_POINT('Ctrl Pts',(0.442467152769555,0.972954924628952,
2.15165128575459));
#22880=CARTESIAN_POINT('Ctrl Pts',(0.490548007340293,1.11648302690173,2.1438007347169));
#22881=CARTESIAN_POINT('Ctrl Pts',(0.636788010918814,1.15554637787772,2.13595018367923));
#22882=CARTESIAN_POINT('Ctrl Pts',(0.750035651880915,1.05511204623542,2.12809963264155));
#22883=CARTESIAN_POINT('Ctrl Pts',(0.728727753027451,0.905251907630433,
2.12024908160387));
#22884=CARTESIAN_POINT('Ctrl Pts',(0.591973745551315,0.840364137654146,
2.11239853056619));
#22885=CARTESIAN_POINT('Ctrl Pts',(0.462417872660985,0.918641551338351,
2.10454797952851));
#22886=CARTESIAN_POINT('Ctrl Pts',(0.456248924787112,1.06988325973025,2.09669742849084));
#22887=CARTESIAN_POINT('Ctrl Pts',(0.578999353953109,1.15845179557081,2.08884687745316));
#22888=CARTESIAN_POINT('Ctrl Pts',(0.720583670983745,1.10491739463527,2.08099632641548));
#22889=CARTESIAN_POINT('Ctrl Pts',(0.754025667034497,0.957289793179509,
2.0731457753778));
#22890=CARTESIAN_POINT('Ctrl Pts',(0.649333818753561,0.847967266182092,
2.06529522434013));
#22891=CARTESIAN_POINT('Ctrl Pts',(0.500398159001457,0.874988272808748,
2.05744467330245));
#22892=CARTESIAN_POINT('Ctrl Pts',(0.440787935610353,1.01412873363258,2.04959412226477));
#22893=CARTESIAN_POINT('Ctrl Pts',(0.523962606599787,1.14058649103877,2.04174357122709));
#22894=CARTESIAN_POINT('Ctrl Pts',(0.675329949855879,1.14098596491627,2.03389302018941));
#22895=CARTESIAN_POINT('Ctrl Pts',(0.759138564770422,1.01490063298166,2.02604246915174));
#22896=CARTESIAN_POINT('Ctrl Pts',(0.700229936626846,0.875541036758072,
2.01819191811406));
#22897=CARTESIAN_POINT('Ctrl Pts',(0.551429170341866,0.847623283599809,
2.01034136707638));
#22898=CARTESIAN_POINT('Ctrl Pts',(0.446190523848043,0.956718572154482,
2.0024908160387));
#22899=CARTESIAN_POINT('Ctrl Pts',(0.468025636826571,1.05475934582637,1.99725711534692));
#22900=CARTESIAN_POINT('Ctrl Pts',(0.497154370004336,1.08857942294107,1.99464026500102));
#22901=CARTESIAN_POINT('Ctrl Pts',(0.567341493646892,0.877840168374445,
2.41607920499693));
#22902=CARTESIAN_POINT('Ctrl Pts',(0.527170074345269,0.888579693265874,
2.41346235465104));
#22903=CARTESIAN_POINT('Ctrl Pts',(0.458901968207183,0.952575032223043,
2.40822865395925));
#22904=CARTESIAN_POINT('Ctrl Pts',(0.482633233158821,1.09178097374987,2.40037810292158));
#22905=CARTESIAN_POINT('Ctrl Pts',(0.611811748491563,1.14840142609121,2.3925275518839));
#22906=CARTESIAN_POINT('Ctrl Pts',(0.730302136799378,1.07206548081067,2.38467700084622));
#22907=CARTESIAN_POINT('Ctrl Pts',(0.731982719715716,0.931032070190328,
2.37682644980854));
#22908=CARTESIAN_POINT('Ctrl Pts',(0.615273515252898,0.85188501296757,2.36897589877086));
#22909=CARTESIAN_POINT('Ctrl Pts',(0.484879152767046,0.905553555365211,
2.36112534773319));
#22910=CARTESIAN_POINT('Ctrl Pts',(0.457721543556091,1.04393279257125,2.35327479669551));
#22911=CARTESIAN_POINT('Ctrl Pts',(0.558165873592863,1.14290753795432,2.34542424565783));
#22912=CARTESIAN_POINT('Ctrl Pts',(0.69612639502905,1.1137217061255,2.33757369462015));
#22913=CARTESIAN_POINT('Ctrl Pts',(0.747879318846525,0.982546373788555,
2.32972314358248));
#22914=CARTESIAN_POINT('Ctrl Pts',(0.667010126969215,0.86702446437302,2.32187259254479));
#22915=CARTESIAN_POINT('Ctrl Pts',(0.526044877463838,0.870757873245112,
2.31402204150712));
#22916=CARTESIAN_POINT('Ctrl Pts',(0.451404229414968,0.99039884837051,2.30617149046944));
#22917=CARTESIAN_POINT('Ctrl Pts',(0.510027857394853,1.11865028592679,2.29832093943177));
#22918=CARTESIAN_POINT('Ctrl Pts',(0.649340613167492,1.14049336632621,2.29047038839408));
#22919=CARTESIAN_POINT('Ctrl Pts',(0.744403548634497,1.03633863539911,2.28261983735641));
#22920=CARTESIAN_POINT('Ctrl Pts',(0.709961941262192,0.899594562711502,
2.27476928631873));
#22921=CARTESIAN_POINT('Ctrl Pts',(0.576903854550442,0.852896467909786,
2.26691873528105));
#22922=CARTESIAN_POINT('Ctrl Pts',(0.464558938233191,0.938124320559086,
2.25906818424337));
#22923=CARTESIAN_POINT('Ctrl Pts',(0.473680787014737,1.07884375217354,2.2512176332057));
#22924=CARTESIAN_POINT('Ctrl Pts',(0.596088708570328,1.14885423313233,2.24336708216801));
#22925=CARTESIAN_POINT('Ctrl Pts',(0.722004369519422,1.08536869865596,2.23551653113034));
#22926=CARTESIAN_POINT('Ctrl Pts',(0.738503611266517,0.945322485882583,
2.22766598009266));
#22927=CARTESIAN_POINT('Ctrl Pts',(0.63078952176059,0.854312367557547,2.21981542905498));
#22928=CARTESIAN_POINT('Ctrl Pts',(0.495462657127491,0.893958381586401,
2.21196487801731));
#22929=CARTESIAN_POINT('Ctrl Pts',(0.453887366832218,1.02870503996507,2.20411432697962));
#22930=CARTESIAN_POINT('Ctrl Pts',(0.543349359582825,1.13770833612116,2.19626377594195));
#22931=CARTESIAN_POINT('Ctrl Pts',(0.683616993454529,1.12321152255188,2.18841322490427));
#22932=CARTESIAN_POINT('Ctrl Pts',(0.748894919716335,0.998215686487819,
2.18056267386659));
#22933=CARTESIAN_POINT('Ctrl Pts',(0.680640342198477,0.874820064977753,
2.17271212282892));
#22934=CARTESIAN_POINT('Ctrl Pts',(0.540065588692086,0.863688785614711,
2.16486157179124));
#22935=CARTESIAN_POINT('Ctrl Pts',(0.453241440086272,0.974804643069725,
2.15701102075356));
#22936=CARTESIAN_POINT('Ctrl Pts',(0.498033857034726,1.10851629728676,2.14916046971588));
#22937=CARTESIAN_POINT('Ctrl Pts',(0.634271935024686,1.14490795296639,2.1413099186782));
#22938=CARTESIAN_POINT('Ctrl Pts',(0.739774127065386,1.05134271792586,2.13345936764053));
#22939=CARTESIAN_POINT('Ctrl Pts',(0.719923558720441,0.911732100097261,
2.12560881660285));
#22940=CARTESIAN_POINT('Ctrl Pts',(0.592522692472719,0.851282258396612,
2.11775826556517));
#22941=CARTESIAN_POINT('Ctrl Pts',(0.471827652244461,0.924205973723485,
2.10990771452749));
#22942=CARTESIAN_POINT('Ctrl Pts',(0.466080622833967,1.06510367037984,2.10205716348981));
#22943=CARTESIAN_POINT('Ctrl Pts',(0.580435670240942,1.14761465778435,2.09420661245214));
#22944=CARTESIAN_POINT('Ctrl Pts',(0.712336482288025,1.09774168382831,2.08635606141445));
#22945=CARTESIAN_POINT('Ctrl Pts',(0.743491249483144,0.960210911204929,
2.07850551037678));
#22946=CARTESIAN_POINT('Ctrl Pts',(0.645959686012189,0.858365379239137,
2.0706549593391));
#22947=CARTESIAN_POINT('Ctrl Pts',(0.507210318313367,0.883538313580547,
2.06280440830142));
#22948=CARTESIAN_POINT('Ctrl Pts',(0.451677071153702,1.01316241430137,2.05495385726375));
#22949=CARTESIAN_POINT('Ctrl Pts',(0.529163101212253,1.13097123127593,2.04710330622607));
#22950=CARTESIAN_POINT('Ctrl Pts',(0.670177840073251,1.13134338357315,2.03925275518839));
#22951=CARTESIAN_POINT('Ctrl Pts',(0.748254456153389,1.01388152043613,2.03140220415071));
#22952=CARTESIAN_POINT('Ctrl Pts',(0.693374819399297,0.884053271842277,
2.02355165311304));
#22953=CARTESIAN_POINT('Ctrl Pts',(0.554751119276,0.858044922970499,2.01570110207535));
#22954=CARTESIAN_POINT('Ctrl Pts',(0.456710155259713,0.959678758219065,
2.00785055103768));
#22955=CARTESIAN_POINT('Ctrl Pts',(0.477051879494498,1.0510141400767,2.00261685034589));
#22956=CARTESIAN_POINT('Ctrl Pts',(0.504188384727762,1.08252112989365,2.));
#22957=CARTESIAN_POINT('Ctrl Pts',(0.473630671680838,1.00010094048498,2.35565803263806));
#22958=CARTESIAN_POINT('Ctrl Pts',(0.473532439388447,1.01274184176985,2.35486362065721));
#22959=CARTESIAN_POINT('Ctrl Pts',(0.475280523076927,1.02535622997532,2.35406920867636));
#22960=CARTESIAN_POINT('Ctrl Pts',(0.478988533430712,1.03736537726742,2.35327479669551));
#22961=CARTESIAN_POINT('Ctrl Pts',(0.491202986901682,1.0769243743656,2.35065794634962));
#22962=CARTESIAN_POINT('Ctrl Pts',(0.524684430247273,1.10991595615996,2.34804109600373));
#22963=CARTESIAN_POINT('Ctrl Pts',(0.564418572159433,1.12154744175234,2.34542424565783));
#22964=CARTESIAN_POINT('Ctrl Pts',(0.604152714071593,1.13317892734471,2.34280739531194));
#22965=CARTESIAN_POINT('Ctrl Pts',(0.650139554550321,1.12345031673511,2.34019054496604));
#22966=CARTESIAN_POINT('Ctrl Pts',(0.681758462092598,1.09672345604081,2.33757369462015));
#22967=CARTESIAN_POINT('Ctrl Pts',(0.713377369634875,1.06999659534652,2.33495684427426));
#22968=CARTESIAN_POINT('Ctrl Pts',(0.7306283442407,1.02627148456754,2.33233999392837));
#22969=CARTESIAN_POINT('Ctrl Pts',(0.725775632897394,0.98515527760879,2.32972314358247));
#22970=CARTESIAN_POINT('Ctrl Pts',(0.720922921554088,0.944039070650043,
2.32710629323658));
#22971=CARTESIAN_POINT('Ctrl Pts',(0.693966524261651,0.905531767511531,
2.32448944289069));
#22972=CARTESIAN_POINT('Ctrl Pts',(0.656994117364537,0.886900350754291,
2.32187259254479));
#22973=CARTESIAN_POINT('Ctrl Pts',(0.620021710467422,0.86826893399705,2.3192557421989));
#22974=CARTESIAN_POINT('Ctrl Pts',(0.57303329396563,0.869513403621081,2.31663889185301));
#22975=CARTESIAN_POINT('Ctrl Pts',(0.537098977706589,0.890075800953996,
2.31402204150712));
#22976=CARTESIAN_POINT('Ctrl Pts',(0.501164661447548,0.910638198286911,
2.31140519116123));
#22977=CARTESIAN_POINT('Ctrl Pts',(0.476284445431258,0.95051852332871,2.30878834081533));
#22978=CARTESIAN_POINT('Ctrl Pts',(0.473614942086427,0.991833925442323,
2.30617149046944));
#22979=CARTESIAN_POINT('Ctrl Pts',(0.4734403457566,0.99453612006154,2.30600033785898));
#22980=CARTESIAN_POINT('Ctrl Pts',(0.4733607599644,0.997244453495218,2.30582918524852));
#22981=CARTESIAN_POINT('Ctrl Pts',(0.473373733146151,0.999953562449677,
2.30565803263806));
#22982=CARTESIAN_POINT('Ctrl Pts',(0.560148615814278,0.850935057178148,
2.4));
#22983=CARTESIAN_POINT('Ctrl Pts',(0.550119440006157,0.854599676739477,
2.4));
#22984=CARTESIAN_POINT('Ctrl Pts',(0.540564996368976,0.859362632124605,
2.4));
#22985=CARTESIAN_POINT('Ctrl Pts',(0.531596820053353,0.865074091447543,
2.4));
#22986=CARTESIAN_POINT('Ctrl Pts',(0.527131647122934,0.867917774785653,
2.4));
#22987=CARTESIAN_POINT('Ctrl Pts',(0.522812231247153,0.870997309268362,
2.4));
#22988=CARTESIAN_POINT('Ctrl Pts',(0.518655594653448,0.874297505825464,
2.4));
#22989=CARTESIAN_POINT('Ctrl Pts',(0.515850253684945,0.876524829864272,
2.4));
#22990=CARTESIAN_POINT('Ctrl Pts',(0.513119107067925,0.878852705294647,
2.4));
#22991=CARTESIAN_POINT('Ctrl Pts',(0.510468112479774,0.881276804671575,
2.4));
#22992=CARTESIAN_POINT('Ctrl Pts',(0.508096911905004,0.883445057244236,
2.4));
#22993=CARTESIAN_POINT('Ctrl Pts',(0.505796540173907,0.885684216423859,
2.4));
#22994=CARTESIAN_POINT('Ctrl Pts',(0.503571411911721,0.887989047157772,
2.4));
#22995=CARTESIAN_POINT('Ctrl Pts',(0.496344342241171,0.895474985193744,
2.4));
#22996=CARTESIAN_POINT('Ctrl Pts',(0.489902891057215,0.903656331605307,
2.4));
#22997=CARTESIAN_POINT('Ctrl Pts',(0.484380306519488,0.912413061717332,
2.4));
#22998=CARTESIAN_POINT('Ctrl Pts',(0.482085857904318,0.91605118932619,2.4));
#22999=CARTESIAN_POINT('Ctrl Pts',(0.479950575517979,0.919788877767087,
2.4));
#23000=CARTESIAN_POINT('Ctrl Pts',(0.477986676370491,0.923618156800881,
2.4));
#23001=CARTESIAN_POINT('Ctrl Pts',(0.476502903437523,0.92651126900086,2.4));
#23002=CARTESIAN_POINT('Ctrl Pts',(0.475117212818011,0.929456979534617,
2.4));
#23003=CARTESIAN_POINT('Ctrl Pts',(0.473840374483033,0.932438138949923,
2.4));
#23004=CARTESIAN_POINT('Ctrl Pts',(0.470678069804683,0.939821481153613,
2.4));
#23005=CARTESIAN_POINT('Ctrl Pts',(0.468171071299299,0.947441891244077,
2.4));
#23006=CARTESIAN_POINT('Ctrl Pts',(0.466390209012142,0.955243589562609,
2.4));
#23007=CARTESIAN_POINT('Ctrl Pts',(0.464752055683344,0.962420100718438,
2.4));
#23008=CARTESIAN_POINT('Ctrl Pts',(0.46372877679908,0.9697505149636,2.4));
#23009=CARTESIAN_POINT('Ctrl Pts',(0.463308980593947,0.977159382735458,
2.4));
#23010=CARTESIAN_POINT('Ctrl Pts',(0.463132836556449,0.980268100410063,
2.4));
#23011=CARTESIAN_POINT('Ctrl Pts',(0.463063518093533,0.983387131233213,
2.4));
#23012=CARTESIAN_POINT('Ctrl Pts',(0.463099417336848,0.986501004293148,
2.4));
#23013=CARTESIAN_POINT('Ctrl Pts',(0.463196741723633,0.994942847577307,
2.4));
#23014=CARTESIAN_POINT('Ctrl Pts',(0.464064109534936,1.00336872849097,2.4));
#23015=CARTESIAN_POINT('Ctrl Pts',(0.46567545593174,1.01166502412979,2.4));
#23016=CARTESIAN_POINT('Ctrl Pts',(0.466871287371351,1.0178219691398,2.4));
#23017=CARTESIAN_POINT('Ctrl Pts',(0.468477485851221,1.02390757093803,2.4));
#23018=CARTESIAN_POINT('Ctrl Pts',(0.47049181446679,1.02987017308613,2.4));
#23019=CARTESIAN_POINT('Ctrl Pts',(0.471677008778134,1.0333784597143,2.4));
#23020=CARTESIAN_POINT('Ctrl Pts',(0.473001300296321,1.03683670710464,2.4));
#23021=CARTESIAN_POINT('Ctrl Pts',(0.474460926720988,1.04022911545352,2.4));
#23022=CARTESIAN_POINT('Ctrl Pts',(0.476751356878834,1.04555244631317,2.4));
#23023=CARTESIAN_POINT('Ctrl Pts',(0.479376309757289,1.05071849279536,2.4));
#23024=CARTESIAN_POINT('Ctrl Pts',(0.482333049272134,1.05568492650343,2.4));
#23025=CARTESIAN_POINT('Ctrl Pts',(0.48437450467299,1.05911395799755,2.4));
#23026=CARTESIAN_POINT('Ctrl Pts',(0.486574676429565,1.06244757032586,2.4));
#23027=CARTESIAN_POINT('Ctrl Pts',(0.4889242778747,1.06565919855071,2.4));
#23028=CARTESIAN_POINT('Ctrl Pts',(0.492216707071327,1.07015956117947,2.4));
#23029=CARTESIAN_POINT('Ctrl Pts',(0.495805971455815,1.07442716938164,2.4));
#23030=CARTESIAN_POINT('Ctrl Pts',(0.499690943915119,1.07842077967776,2.4));
#23031=CARTESIAN_POINT('Ctrl Pts',(0.501092720341441,1.07986175482692,2.4));
#23032=CARTESIAN_POINT('Ctrl Pts',(0.502533036573698,1.08126699616446,2.4));
#23033=CARTESIAN_POINT('Ctrl Pts',(0.504010178078511,1.08263575731582,2.4));
#23034=CARTESIAN_POINT('Origin',(-0.6,1.,2.15));
#23035=CARTESIAN_POINT('Origin',(0.6,1.,2.15));
#23036=CARTESIAN_POINT('Origin',(0.,0.,7.8));
#23037=CARTESIAN_POINT('',(-0.6,-0.2,7.8));
#23038=CARTESIAN_POINT('Origin',(-0.6,0.,7.8));
#23039=CARTESIAN_POINT('',(-1.,-0.2,7.8));
#23040=CARTESIAN_POINT('',(0.,-0.2,7.8));
#23041=CARTESIAN_POINT('Origin',(-1.,0.,7.8));
#23042=CARTESIAN_POINT('Origin',(0.,0.,7.8));
#23043=CARTESIAN_POINT('',(1.,-0.2,7.8));
#23044=CARTESIAN_POINT('Origin',(1.,0.,7.8));
#23045=CARTESIAN_POINT('',(0.6,-0.2,7.8));
#23046=CARTESIAN_POINT('',(0.,-0.2,7.8));
#23047=CARTESIAN_POINT('Origin',(0.6,0.,7.8));
#23048=CARTESIAN_POINT('Origin',(0.6,0.6,6.8));
#23049=CARTESIAN_POINT('',(0.6,-0.6,7.));
#23050=CARTESIAN_POINT('',(0.6,0.6,7.));
#23051=CARTESIAN_POINT('',(0.6,0.3,7.));
#23052=CARTESIAN_POINT('',(0.6,-0.6,8.6));
#23053=CARTESIAN_POINT('',(0.6,-0.6,6.8));
#23054=CARTESIAN_POINT('',(0.6,0.6,8.6));
#23055=CARTESIAN_POINT('',(0.6,0.6,8.6));
#23056=CARTESIAN_POINT('',(0.6,0.6,6.8));
#23057=CARTESIAN_POINT('Origin',(0.8,0.,8.6));
#23058=CARTESIAN_POINT('',(1.,-0.6,8.6));
#23059=CARTESIAN_POINT('',(0.6,-0.6,8.6));
#23060=CARTESIAN_POINT('',(1.,0.6,8.6));
#23061=CARTESIAN_POINT('',(1.,-0.6,8.6));
#23062=CARTESIAN_POINT('',(1.,0.6,8.6));
#23063=CARTESIAN_POINT('Origin',(-1.,-0.6,6.6));
#23064=CARTESIAN_POINT('',(1.,-0.6,6.6));
#23065=CARTESIAN_POINT('',(1.,-0.6,6.6));
#23066=CARTESIAN_POINT('',(-0.6,-0.6,7.));
#23067=CARTESIAN_POINT('',(-1.,-0.6,7.));
#23068=CARTESIAN_POINT('',(-0.6,-0.6,8.6));
#23069=CARTESIAN_POINT('',(-0.6,-0.6,6.8));
#23070=CARTESIAN_POINT('',(-1.,-0.6,8.6));
#23071=CARTESIAN_POINT('',(-1.,-0.6,8.6));
#23072=CARTESIAN_POINT('',(-1.,-0.6,6.6));
#23073=CARTESIAN_POINT('',(-1.,-0.6,6.6));
#23074=CARTESIAN_POINT('',(0.,-0.6,6.6));
#23075=CARTESIAN_POINT('',(-1.,-0.6,6.6));
#23076=CARTESIAN_POINT('',(-1.,-0.6,6.6));
#23077=CARTESIAN_POINT('Origin',(0.,0.,7.));
#23078=CARTESIAN_POINT('',(-0.6,0.6,7.));
#23079=CARTESIAN_POINT('',(1.,0.6,7.));
#23080=CARTESIAN_POINT('',(-0.6,-0.3,7.));
#23081=CARTESIAN_POINT('Origin',(-0.6,-0.6,6.8));
#23082=CARTESIAN_POINT('',(-0.6,0.6,8.6));
#23083=CARTESIAN_POINT('',(-0.6,0.6,6.8));
#23084=CARTESIAN_POINT('',(-0.6,-0.6,8.6));
#23085=CARTESIAN_POINT('Origin',(-0.8,0.,8.6));
#23086=CARTESIAN_POINT('',(-1.,0.6,8.6));
#23087=CARTESIAN_POINT('',(-1.,0.6,8.6));
#23088=CARTESIAN_POINT('',(-0.6,0.6,8.6));
#23089=CARTESIAN_POINT('Origin',(0.,0.,6.6));
#23090=CARTESIAN_POINT('',(0.,0.6,6.6));
#23091=CARTESIAN_POINT('Origin',(0.,0.,6.6));
#23092=CARTESIAN_POINT('',(1.,0.6,6.6));
#23093=CARTESIAN_POINT('',(1.,0.6,6.6));
#23094=CARTESIAN_POINT('',(1.,-0.6,6.6));
#23095=CARTESIAN_POINT('Origin',(0.,0.,6.6));
#23096=CARTESIAN_POINT('',(-0.6,-7.34788079488412E-17,6.6));
#23097=CARTESIAN_POINT('Origin',(0.,0.,6.6));
#23098=CARTESIAN_POINT('',(-1.,0.6,6.6));
#23099=CARTESIAN_POINT('',(-1.,0.6,6.6));
#23100=CARTESIAN_POINT('',(1.,0.6,6.6));
#23101=CARTESIAN_POINT('Origin',(0.,0.,6.6));
#23102=CARTESIAN_POINT('Origin',(1.,0.6,6.6));
#23103=CARTESIAN_POINT('',(1.,0.6,6.6));
#23104=CARTESIAN_POINT('',(-1.,0.6,6.6));
#23105=CARTESIAN_POINT('Origin',(1.,-0.6,6.6));
#23106=CARTESIAN_POINT('Origin',(-1.,0.6,6.6));
#23107=CARTESIAN_POINT('Origin',(-1.8,0.6,2.));
#23108=CARTESIAN_POINT('',(0.8,0.6,2.4));
#23109=CARTESIAN_POINT('',(0.8,0.6,2.));
#23110=CARTESIAN_POINT('',(1.8,0.6,2.4));
#23111=CARTESIAN_POINT('',(1.8,0.6,2.));
#23112=CARTESIAN_POINT('',(-1.8,0.6,2.4));
#23113=CARTESIAN_POINT('Origin',(1.8,1.4,2.));
#23114=CARTESIAN_POINT('',(-1.8,1.4,2.4));
#23115=CARTESIAN_POINT('',(-1.8,1.4,2.));
#23116=CARTESIAN_POINT('',(1.8,1.4,2.4));
#23117=CARTESIAN_POINT('',(1.8,1.4,2.4));
#23118=CARTESIAN_POINT('',(1.8,1.4,2.));
#23119=CARTESIAN_POINT('Origin',(1.8,0.6,2.));
#23120=CARTESIAN_POINT('',(1.8,0.6,2.4));
#23121=CARTESIAN_POINT('Origin',(-1.8,0.6,2.));
#23122=CARTESIAN_POINT('',(-0.8,0.6,2.4));
#23123=CARTESIAN_POINT('',(-0.8,0.6,2.));
#23124=CARTESIAN_POINT('',(-1.8,0.6,2.4));
#23125=CARTESIAN_POINT('',(-1.8,0.6,2.4));
#23126=CARTESIAN_POINT('',(-1.8,0.6,2.));
#23127=CARTESIAN_POINT('Origin',(-1.8,1.4,2.));
#23128=CARTESIAN_POINT('',(-1.8,1.4,2.4));
#23129=CARTESIAN_POINT('Origin',(0.,0.,2.));
#23130=CARTESIAN_POINT('Origin',(0.,0.,2.4));
#23131=CARTESIAN_POINT('Origin',(0.,0.,2.4));
#23132=CARTESIAN_POINT('',(-0.6,-7.34788079488412E-17,2.4));
#23133=CARTESIAN_POINT('',(-0.6,-7.34788079488412E-17,2.4));
#23134=CARTESIAN_POINT('Origin',(0.,0.,2.4));
#23135=CARTESIAN_POINT('Origin',(0.,0.,2.4));
#36449=UNCERTAINTY_MEASURE_WITH_UNIT(LENGTH_MEASURE(0.001),#36483,
'DISTANCE_ACCURACY_VALUE',
'Maximum model space distance between geometric entities at asserted c
onnectivities');
#36463=UNCERTAINTY_MEASURE_WITH_UNIT(LENGTH_MEASURE(0.001),#36483,
'DISTANCE_ACCURACY_VALUE',
'Maximum model space distance between geometric entities at asserted c
onnectivities');
#36468=(
GEOMETRIC_REPRESENTATION_CONTEXT(3)
GLOBAL_UNCERTAINTY_ASSIGNED_CONTEXT((#36449))
GLOBAL_UNIT_ASSIGNED_CONTEXT((#36483,#36485,#36486))
REPRESENTATION_CONTEXT('','3D')
);
#36482=(
GEOMETRIC_REPRESENTATION_CONTEXT(3)
GLOBAL_UNCERTAINTY_ASSIGNED_CONTEXT((#36463))
GLOBAL_UNIT_ASSIGNED_CONTEXT((#36483,#36485,#36486))
REPRESENTATION_CONTEXT('','3D')
);
#36483=(
LENGTH_UNIT()
NAMED_UNIT(*)
SI_UNIT(.CENTI.,.METRE.)
);
#36485=(
NAMED_UNIT(*)
PLANE_ANGLE_UNIT()
SI_UNIT($,.RADIAN.)
);
#36486=(
NAMED_UNIT(*)
SI_UNIT($,.STERADIAN.)
SOLID_ANGLE_UNIT()
);
#36491=SHAPE_DEFINITION_REPRESENTATION(#36509,#36558);
#36509=PRODUCT_DEFINITION_SHAPE('',$,#36577);
#36558=SHAPE_REPRESENTATION('',(#10207),#36468);
#36572=PRODUCT_DEFINITION_CONTEXT('part definition',#36628,'design');
#36577=PRODUCT_DEFINITION('Roller actuator','Roller actuator',#36595,#36572);
#36595=PRODUCT_DEFINITION_FORMATION('',$,#36634);
#36628=APPLICATION_CONTEXT(
'Core Data for Automotive Mechanical Design Process');
#36629=PRODUCT_CONTEXT('part definition',#36628,'mechanical');
#36634=PRODUCT('Roller actuator','Roller actuator',$,(#36629));
#36652=PRESENTATION_STYLE_ASSIGNMENT((#36666));
#36666=SURFACE_STYLE_USAGE(.BOTH.,#36680);
#36680=SURFACE_SIDE_STYLE('',(#36694));
#36694=SURFACE_STYLE_FILL_AREA(#36708);
#36708=FILL_AREA_STYLE('Light blue',(#36722));
#36722=FILL_AREA_STYLE_COLOUR('Light blue',#36736);
#36736=COLOUR_RGB('Light blue',0.662745098039216,0.831372549019608,0.949019607843137);
ENDSEC;
END-ISO-10303-21;
